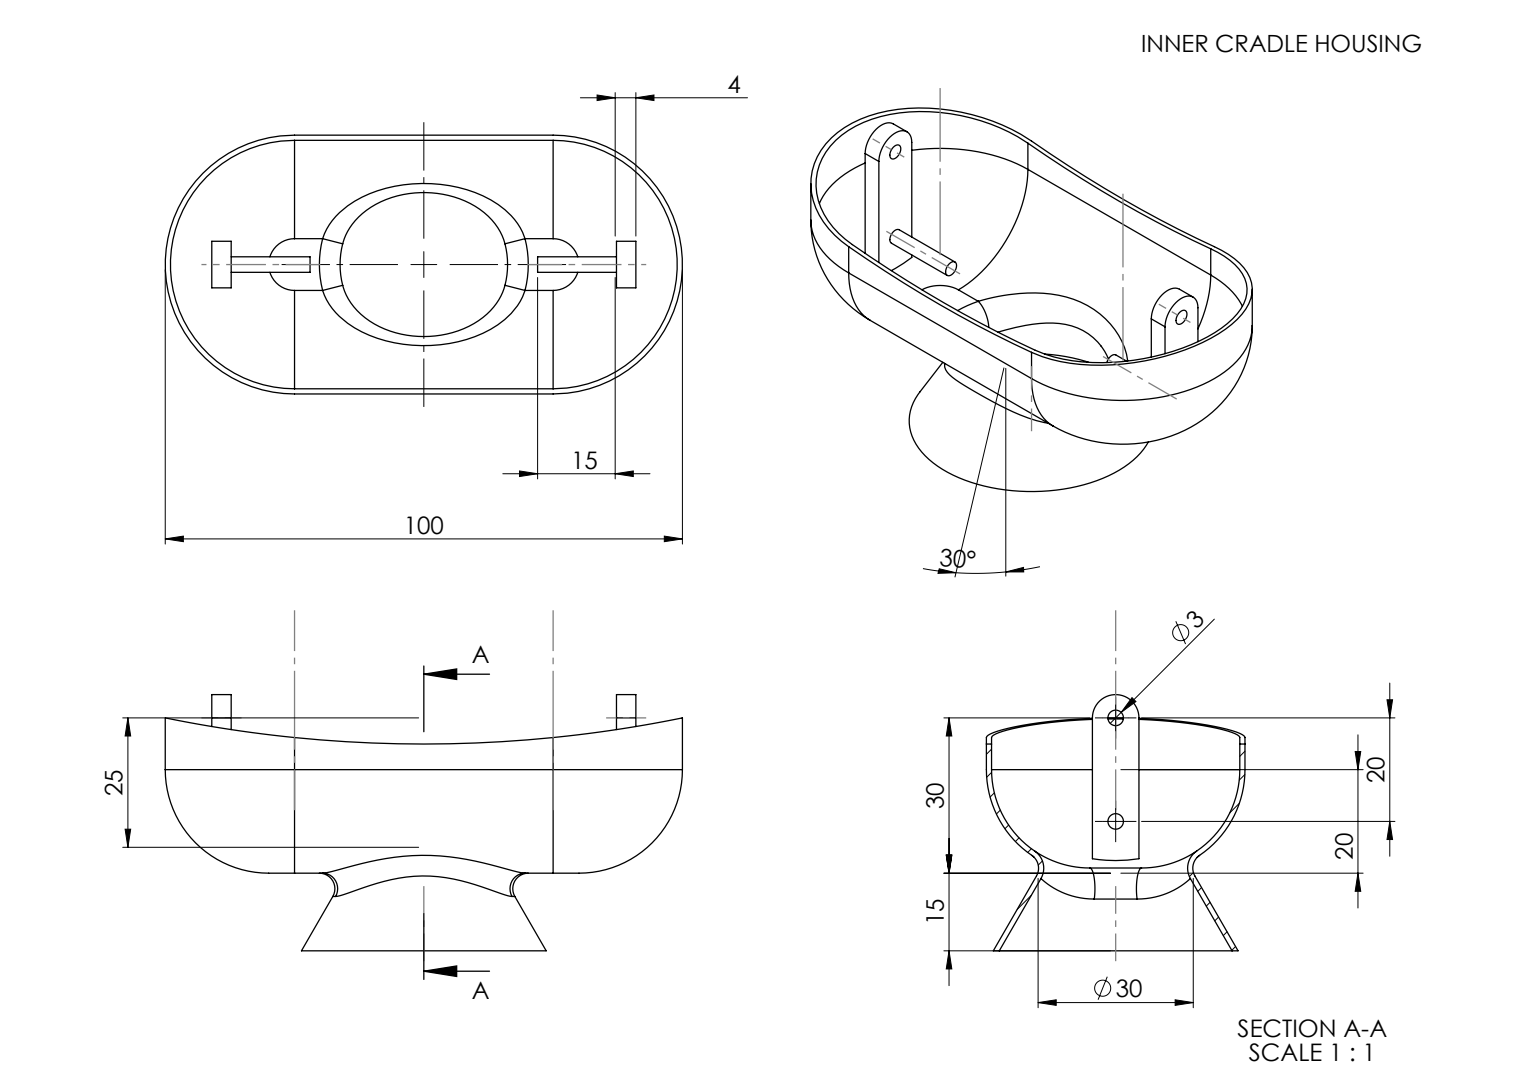
ISO-10303-21;
HEADER;
FILE_DESCRIPTION (('STEP AP214'),
    '1' );
FILE_NAME ('Inner cradle housing.step',
    '2026-10-09T15:17:24',
    ( '' ),
    ( '' ),
    'SwSTEP 2.0',
    'SolidWorks 2026',
    '' );
FILE_SCHEMA (( 'AUTOMOTIVE_DESIGN' ));
ENDSEC;

DATA;
#11=EDGE_LOOP ( 'NONE', ( #13476, #2905, #46275, #26509, #7082, #64281 ) ) ;
#18=CARTESIAN_POINT ( 'NONE',  ( -9.857630741398541119, -27.64257788600498245, 14.42778837489968424 ) ) ;
#57=CARTESIAN_POINT ( 'NONE',  ( 1.074417311476297821, -26.55384113566742599, -16.22365110280896161 ) ) ;
#110=CARTESIAN_POINT ( 'NONE',  ( 49.33927601438018229, -0.1339636383559821564, -5.724480317196142032 ) ) ;
#114=CARTESIAN_POINT ( 'NONE',  ( -38.20713125073509531, -2.115151932665340961, -21.24219930640693832 ) ) ;
#116=CARTESIAN_POINT ( 'NONE',  ( 19.56743653832046803, -28.99999999999999645, -5.000000000000000888 ) ) ;
#121=ADVANCED_FACE ( 'NONE', ( #65020 ), #19493, .F. ) ;
#146=DIRECTION ( 'NONE',  ( 1.000000000000000000, 0.000000000000000000, 0.000000000000000000 ) ) ;
#147=CARTESIAN_POINT ( 'NONE',  ( -8.315422948566315142, -32.37591480791618892, 12.77210737139424523 ) ) ;
#159=CARTESIAN_POINT ( 'NONE',  ( 14.19127861764911813, -30.11167671974727611, 5.095448428665359408 ) ) ;
#215=CARTESIAN_POINT ( 'NONE',  ( 16.21117406328132304, -34.99999999999999289, -4.142385751841744401 ) ) ;
#249=CARTESIAN_POINT ( 'NONE',  ( -41.00000000000000711, -1.694065894508600678E-18, 0.000000000000000000 ) ) ;
#284=FACE_OUTER_BOUND ( 'NONE', #48979, .T. ) ;
#285=CYLINDRICAL_SURFACE ( 'NONE', #47961, 1.500000000000000222 ) ;
#326=FACE_OUTER_BOUND ( 'NONE', #43910, .T. ) ;
#391=CARTESIAN_POINT ( 'NONE',  ( 36.99853283657033387, -2.301590494557431477, -20.84413141647362266 ) ) ;
#412=CARTESIAN_POINT ( 'NONE',  ( -5.808548865028119401, -28.57390223679843544, -12.95295593664668310 ) ) ;
#426=CARTESIAN_POINT ( 'NONE',  ( 25.00000000000000711, -30.00000000000000000, -24.00000000000000000 ) ) ;
#465=CARTESIAN_POINT ( 'NONE',  ( 15.59244419633153456, -34.16973227397373591, 7.752328951095602605 ) ) ;
#491=CARTESIAN_POINT ( 'NONE',  ( -12.26308380404417164, -33.73908083898199806, 10.29207979367737380 ) ) ;
#501=CARTESIAN_POINT ( 'NONE',  ( 10.20102756488484275, -27.72270395345634952, 14.27139701651698722 ) ) ;
#542=CARTESIAN_POINT ( 'NONE',  ( -15.05999060605171458, -34.74914171045087841, -6.965575872675125346 ) ) ;
#548=CARTESIAN_POINT ( 'NONE',  ( 15.30590914263659386, -28.05839919878968303, -10.93630420992710128 ) ) ;
#556=B_SPLINE_CURVE_WITH_KNOTS ( 'NONE', 3,
 ( #63039, #7858, #51545, #7500, #658, #6873, #56507, #1875, #12169, #47438, #22145, #2879, #2553, #27143, #33103, #23135, #10952, #42744, #32440, #62695, #52750, #63355, #20917, #31239, #5658, #61474, #28134, #48097, #22822, #32755, #17162, #37439, #43078, #12481, #18153, #53412, #27793, #25927, #47754, #17821, #57750, #46216, #33445, #17503, #15916, #37773, #53064, #2203, #7174, #36200, #38426, #41191, #22481, #38086 ),
 .UNSPECIFIED., .F., .F.,
 ( 4, 2, 2, 2, 2, 2, 2, 2, 2, 2, 2, 2, 2, 2, 2, 2, 2, 2, 2, 2, 2, 2, 2, 2, 2, 2, 4 ),
 ( 0.000000000000000000, 0.004712545709777801912, 0.007068818564666702435, 0.009425091419555603825, 0.01413763712933342048, 0.01649390998422233315, 0.01885018283911124234, 0.02356272854888905727, 0.02591900140377796299, 0.02827527425866686525, 0.03063154711355577098, 0.03180968354100022211, 0.03298781996844467324, 0.03770036567822248469, 0.04005663853311138001, 0.04123477496055583114, 0.04241291138800028920, 0.04712545709777810760, 0.04948172995266700985, 0.05183800280755592599, 0.05655054851733373744, 0.06126309422711155583, 0.06361936708200047197, 0.06597563993688937423, 0.07068818564666717874, 0.07304445850155608100, 0.07540073135644498326 ),
 .UNSPECIFIED. ) ;
#623=AXIS2_PLACEMENT_3D ( 'NONE', #44497, #64774, #4635 ) ;
#631=EDGE_CURVE ( 'NONE', #31040, #33343, #47243, .T. ) ;
#637=ORIENTED_EDGE ( 'NONE', *, *, #44495, .F. ) ;
#653=CARTESIAN_POINT ( 'NONE',  ( -17.92531974009704498, -29.71422580122558088, 8.391737566679434934 ) ) ;
#658=CARTESIAN_POINT ( 'NONE',  ( -31.19808003874556235, -3.097905286366202215, 23.19915556217947739 ) ) ;
#659=VERTEX_POINT ( 'NONE', #32553 ) ;
#690=CARTESIAN_POINT ( 'NONE',  ( -4.968020780095184108, -25.99038707641916091, -15.26464785194325913 ) ) ;
#713=LINE ( 'NONE', #60899, #29959 ) ;
#727=CARTESIAN_POINT ( 'NONE',  ( 18.66975156949926529, -29.88417193384192316, -7.188590896528729068 ) ) ;
#769=CARTESIAN_POINT ( 'NONE',  ( 49.19530910174992044, -0.1631003452855546987, 6.502801691937079021 ) ) ;
#773=CARTESIAN_POINT ( 'NONE',  ( 3.657075258475105617, -30.77912794045789724, 15.01778408663561493 ) ) ;
#799=CARTESIAN_POINT ( 'NONE',  ( 3.702144525957873356, -25.87585389521097312, 15.43847573974272613 ) ) ;
#850=CARTESIAN_POINT ( 'NONE',  ( 11.32672149592540833, -33.39346531321398714, 11.05302976539647197 ) ) ;
#856=CARTESIAN_POINT ( 'NONE',  ( 9.730232070128172595, -26.74067542416307219, -13.98809302346541372 ) ) ;
#889=EDGE_CURVE ( 'NONE', #27125, #49767, #43081, .T. ) ;
#939=VERTEX_POINT ( 'NONE', #30517 ) ;
#971=CARTESIAN_POINT ( 'NONE',  ( 41.00000000000000711, -25.03188948156373783, 4.499999999999997335 ) ) ;
#990=CARTESIAN_POINT ( 'NONE',  ( -17.07517663476617997, -28.52001404462332701, 9.261390606240922807 ) ) ;
#1000=FACE_OUTER_BOUND ( 'NONE', #53126, .T. ) ;
#1013=CARTESIAN_POINT ( 'NONE',  ( 7.856790134851108220, -26.39165916151114999, -14.61432118582568407 ) ) ;
#1036=CARTESIAN_POINT ( 'NONE',  ( 46.86486279825821555, -0.6193039491651846085, 9.927184253397724589 ) ) ;
#1044=CARTESIAN_POINT ( 'NONE',  ( 2.756135405615951955E-15, -45.00000000000000000, 22.50555349946515804 ) ) ;
#1054=CARTESIAN_POINT ( 'NONE',  ( 9.591596427418878079, -32.12122108032075118, -13.09346764506430993 ) ) ;
#1064=CARTESIAN_POINT ( 'NONE',  ( -4.348075857607831551, -31.41176936172747958, 14.02665938297152870 ) ) ;
#1072=AXIS2_PLACEMENT_3D ( 'NONE', #24249, #60472, #45192 ) ;
#1108=CIRCLE ( 'NONE', #30794, 3.999999999999999112 ) ;
#1130=CARTESIAN_POINT ( 'NONE',  ( 8.754896909465220034, -28.78086681028207749, 9.883947858767236028 ) ) ;
#1134=CYLINDRICAL_SURFACE ( 'NONE', #47965, 20.00000000000000000 ) ;
#1145=ORIENTED_EDGE ( 'NONE', *, *, #50067, .F. ) ;
#1159=CARTESIAN_POINT ( 'NONE',  ( 25.00000000000000355, -28.99999999999999645, -4.999999999999999112 ) ) ;
#1164=DIRECTION ( 'NONE',  ( 0.000000000000000000, -0.000000000000000000, 1.000000000000000000 ) ) ;
#1172=CIRCLE ( 'NONE', #59553, 1.500000000000000222 ) ;
#1234=VECTOR ( 'NONE', #2454, 1000.000000000000000 ) ;
#1256=FACE_BOUND ( 'NONE', #34167, .T. ) ;
#1266=DIRECTION ( 'NONE',  ( 0.000000000000000000, 0.000000000000000000, 1.000000000000000000 ) ) ;
#1314=ORIENTED_EDGE ( 'NONE', *, *, #9225, .T. ) ;
#1316=CARTESIAN_POINT ( 'NONE',  ( -19.56743653832047158, -33.00000000000000000, 5.000000000000000888 ) ) ;
#1323=EDGE_LOOP ( 'NONE', ( #39107, #2329, #36527, #17256 ) ) ;
#1346=ORIENTED_EDGE ( 'NONE', *, *, #6034, .T. ) ;
#1350=CARTESIAN_POINT ( 'NONE',  ( 9.722110222095126986, -26.73349363795548328, -14.00621188957225272 ) ) ;
#1357=CARTESIAN_POINT ( 'NONE',  ( -19.56743653832047514, -30.00000000000000000, 5.000000000000000888 ) ) ;
#1395=CARTESIAN_POINT ( 'NONE',  ( 19.43600551875691451, -29.99999999999999645, -5.447264023289523749 ) ) ;
#1397=ORIENTED_EDGE ( 'NONE', *, *, #11958, .F. ) ;
#1476=CARTESIAN_POINT ( 'NONE',  ( 3.024435290549866817, -27.93754772256033192, 12.30283293119135202 ) ) ;
#1547=EDGE_CURVE ( 'NONE', #54224, #31440, #12444, .T. ) ;
#1551=LINE ( 'NONE', #37087, #27003 ) ;
#1610=CARTESIAN_POINT ( 'NONE',  ( -49.33927601438018939, -0.1339636383559742183, 5.724480317196145585 ) ) ;
#1683=CARTESIAN_POINT ( 'NONE',  ( -0.4967434119545894866, -25.72578597719286364, -15.66300405139958407 ) ) ;
#1702=CARTESIAN_POINT ( 'NONE',  ( 48.61333473403966821, -0.2789806315675412152, 4.308813575818149388 ) ) ;
#1709=ADVANCED_FACE ( 'NONE', ( #31357 ), #52315, .T. ) ;
#1718=CARTESIAN_POINT ( 'NONE',  ( 9.992127424267872371, -32.24574823824523406, -12.88148438038769150 ) ) ;
#1725=CARTESIAN_POINT ( 'NONE',  ( 16.21117406328131594, -35.00000000000000000, -4.142385751841773711 ) ) ;
#1730=FACE_OUTER_BOUND ( 'NONE', #16630, .T. ) ;
#1736=EDGE_CURVE ( 'NONE', #3747, #26969, #6009, .T. ) ;
#1788=DIRECTION ( 'NONE',  ( -0.9688695217174486674, 0.000000000000000000, -0.2475719085175094036 ) ) ;
#1792=CARTESIAN_POINT ( 'NONE',  ( 5.926183177043330197, -31.73296902231061978, 13.63811545878544607 ) ) ;
#1799=EDGE_CURVE ( 'NONE', #65150, #23145, #39949, .T. ) ;
#1810=DIRECTION ( 'NONE',  ( 0.000000000000000000, 1.000000000000000000, 0.000000000000000000 ) ) ;
#1813=DIRECTION ( 'NONE',  ( 0.000000000000000000, 0.000000000000000000, -1.000000000000000000 ) ) ;
#1827=EDGE_CURVE ( 'NONE', #7333, #31040, #33603, .T. ) ;
#1875=CARTESIAN_POINT ( 'NONE',  ( -35.62380706382417372, -2.504225566391070856, 21.57767586339570443 ) ) ;
#1923=CARTESIAN_POINT ( 'NONE',  ( -12.81094353615575088, -29.07674955874293943, -3.635823793966369788 ) ) ;
#2014=CARTESIAN_POINT ( 'NONE',  ( 31.24126863879125438, -3.096129103239020797, 23.22707964006411530 ) ) ;
#2031=CARTESIAN_POINT ( 'NONE',  ( 8.782331025771476618, -31.88110954670732866, -13.48440172003491178 ) ) ;
#2037=DIRECTION ( 'NONE',  ( 0.000000000000000000, 0.000000000000000000, 1.000000000000000000 ) ) ;
#2072=CARTESIAN_POINT ( 'NONE',  ( 19.24109636373441390, -29.98159021036885363, -5.977446804020350335 ) ) ;
#2100=DIRECTION ( 'NONE',  ( 0.000000000000000000, 0.000000000000000000, 1.000000000000000000 ) ) ;
#2108=CARTESIAN_POINT ( 'NONE',  ( 13.74768401152558894, -27.65692779101644305, 12.04119239038937117 ) ) ;
#2140=DIRECTION ( 'NONE',  ( 0.000000000000000000, -1.000000000000000000, 0.000000000000000000 ) ) ;
#2158=LINE ( 'NONE', #52714, #51393 ) ;
#2178=VECTOR ( 'NONE', #11059, 1000.000000000000000 ) ;
#2201=CARTESIAN_POINT ( 'NONE',  ( -15.83540182711247191, -34.24586518154816872, 7.348477566591424370 ) ) ;
#2203=CARTESIAN_POINT ( 'NONE',  ( -32.73308617475133531, -2.903166307960748593, -22.77405829473930865 ) ) ;
#2252=CIRCLE ( 'NONE', #10729, 1.500000000000000222 ) ;
#2259=CARTESIAN_POINT ( 'NONE',  ( -12.58725039716645000, -33.86007533429943095, -10.00564543523592320 ) ) ;
#2269=VERTEX_POINT ( 'NONE', #41398 ) ;
#2273=AXIS2_PLACEMENT_3D ( 'NONE', #3939, #24202, #8262 ) ;
#2295=CARTESIAN_POINT ( 'NONE',  ( -14.80332308495361815, -33.90539544391017301, -8.876538241604327695 ) ) ;
#2310=FACE_BOUND ( 'NONE', #52616, .T. ) ;
#2329=ORIENTED_EDGE ( 'NONE', *, *, #24038, .F. ) ;
#2344=AXIS2_PLACEMENT_3D ( 'NONE', #27897, #6645, #37868 ) ;
#2349=CARTESIAN_POINT ( 'NONE',  ( -8.868684597663976987, -31.89901926473304883, 13.46243262195112678 ) ) ;
#2361=CARTESIAN_POINT ( 'NONE',  ( 25.79281180259795292, -3.718204414137759262, 24.00000000000000355 ) ) ;
#2384=ORIENTED_EDGE ( 'NONE', *, *, #27450, .F. ) ;
#2421=CARTESIAN_POINT ( 'NONE',  ( 9.836964722002395689, -27.64452029744604644, -14.41904541651817873 ) ) ;
#2441=ORIENTED_EDGE ( 'NONE', *, *, #38364, .T. ) ;
#2454=DIRECTION ( 'NONE',  ( 6.123233995736778362E-17, -0.8660254037844380415, 0.5000000000000009992 ) ) ;
#2553=CARTESIAN_POINT ( 'NONE',  ( -41.38732981120779186, -1.602042930228848583, 17.55180477253565030 ) ) ;
#2561=AXIS2_PLACEMENT_3D ( 'NONE', #19143, #40066, #50410 ) ;
#2583=DIRECTION ( 'NONE',  ( -1.000000000000000000, 0.000000000000000000, 0.000000000000000000 ) ) ;
#2611=CARTESIAN_POINT ( 'NONE',  ( -13.20530710592869283, -34.09051099065911217, -9.405657446765959051 ) ) ;
#2646=ORIENTED_EDGE ( 'NONE', *, *, #13071, .F. ) ;
#2649=ORIENTED_EDGE ( 'NONE', *, *, #13071, .T. ) ;
#2723=ORIENTED_EDGE ( 'NONE', *, *, #63965, .F. ) ;
#2766=CARTESIAN_POINT ( 'NONE',  ( 2.022082860508893187, -26.59007814299271999, -16.17076096363556914 ) ) ;
#2786=VECTOR ( 'NONE', #40970, 1000.000000000000000 ) ;
#2839=CARTESIAN_POINT ( 'NONE',  ( 16.93394556191337230, -34.50000000000000000, 4.811904876957209254 ) ) ;
#2865=DIRECTION ( 'NONE',  ( 0.000000000000000000, 0.000000000000000000, 1.000000000000000000 ) ) ;
#2875=CARTESIAN_POINT ( 'NONE',  ( -7.049735699850023352, -28.78059498260736504, 12.46475915493964415 ) ) ;
#2879=CARTESIAN_POINT ( 'NONE',  ( -40.80553070818748296, -1.699139512677864561, 18.07784515657014168 ) ) ;
#2905=ORIENTED_EDGE ( 'NONE', *, *, #10978, .T. ) ;
#2914=CARTESIAN_POINT ( 'NONE',  ( -49.59714883329487378, -0.08190040965286676800, -4.488761805454715592 ) ) ;
#2956=DIRECTION ( 'NONE',  ( 0.000000000000000000, 0.000000000000000000, 1.000000000000000000 ) ) ;
#2963=ORIENTED_EDGE ( 'NONE', *, *, #9225, .F. ) ;
#2970=FACE_OUTER_BOUND ( 'NONE', #29494, .T. ) ;
#2994=DIRECTION ( 'NONE',  ( -0.000000000000000000, -1.000000000000000000, -0.000000000000000000 ) ) ;
#3000=CARTESIAN_POINT ( 'NONE',  ( 16.78995969943013478, -34.48221411999237773, -5.258039666742740259 ) ) ;
#3020=ORIENTED_EDGE ( 'NONE', *, *, #57969, .F. ) ;
#3040=ORIENTED_EDGE ( 'NONE', *, *, #50249, .F. ) ;
#3123=EDGE_CURVE ( 'NONE', #46997, #34941, #52958, .T. ) ;
#3139=AXIS2_PLACEMENT_3D ( 'NONE', #59983, #46975, #61929 ) ;
#3193=CARTESIAN_POINT ( 'NONE',  ( -6.227954140665750593, -28.64022186353238553, 12.80077302199559419 ) ) ;
#3209=CARTESIAN_POINT ( 'NONE',  ( 25.00000000000000355, -9.999999999999998224, 1.530808498934191521E-15 ) ) ;
#3214=DIRECTION ( 'NONE',  ( 0.000000000000000000, 0.000000000000000000, -1.000000000000000000 ) ) ;
#3223=DIRECTION ( 'NONE',  ( -1.000000000000000000, -0.000000000000000000, 0.000000000000000000 ) ) ;
#3248=CARTESIAN_POINT ( 'NONE',  ( 4.261270162784661863, -31.40576903066106240, -14.03034928007075344 ) ) ;
#3255=LINE ( 'NONE', #17561, #52176 ) ;
#3280=DIRECTION ( 'NONE',  ( 1.000000000000000000, -0.000000000000000000, -0.000000000000000000 ) ) ;
#3285=CYLINDRICAL_SURFACE ( 'NONE', #63068, 1.500000000000000444 ) ;
#3299=AXIS2_PLACEMENT_3D ( 'NONE', #41370, #36726, #26420 ) ;
#3329=CARTESIAN_POINT ( 'NONE',  ( 14.80527133490444314, -33.90607016887765468, -8.874040421132026069 ) ) ;
#3387=ORIENTED_EDGE ( 'NONE', *, *, #9032, .F. ) ;
#3397=AXIS2_PLACEMENT_3D ( 'NONE', #54729, #14943, #35571 ) ;
#3414=CARTESIAN_POINT ( 'NONE',  ( 19.56743653832047158, -30.00000000000000000, -5.000000000000000888 ) ) ;
#3444=AXIS2_PLACEMENT_3D ( 'NONE', #65419, #19888, #55799 ) ;
#3457=B_SPLINE_CURVE_WITH_KNOTS ( 'NONE', 3,
 ( #15365, #6066, #45617, #51294, #35307, #41938, #1064, #56250, #6381, #10692, #46295, #55620, #41613, #61900, #46943, #16359, #36633, #56937, #11355, #5077, #20689, #50952, #5400, #21683, #35639, #62225 ),
 .UNSPECIFIED., .F., .F.,
 ( 4, 2, 2, 2, 2, 2, 2, 2, 2, 2, 2, 2, 4 ),
 ( 0.02137397820462155415, 0.02270922547143531048, 0.02404447273824906334, 0.02671496727187657599, 0.02805021453869033232, 0.02938546180550408865, 0.03205595633913160825, 0.03472645087275912090, 0.03606169813957287723, 0.03739694540638663356, 0.03873219267320038989, 0.04006743994001414622, 0.04273793447364165887 ),
 .UNSPECIFIED. ) ;
#3533=VECTOR ( 'NONE', #14513, 1000.000000000000000 ) ;
#3536=CARTESIAN_POINT ( 'NONE',  ( -11.13200843151504849, -27.92871652161695550, 13.87829993151233943 ) ) ;
#3594=CARTESIAN_POINT ( 'NONE',  ( -0.4223990570890304164, -27.81390085543024426, -12.58355210400658564 ) ) ;
#3606=CYLINDRICAL_SURFACE ( 'NONE', #18532, 4.500000000000000888 ) ;
#3650=CARTESIAN_POINT ( 'NONE',  ( -16.66082797316812503, -33.00000000000000000, 4.257284274447473926 ) ) ;
#3718=CARTESIAN_POINT ( 'NONE',  ( -15.84367078532069861, -34.24835312396456999, -7.333865081863226720 ) ) ;
#3747=VERTEX_POINT ( 'NONE', #11496 ) ;
#3768=EDGE_LOOP ( 'NONE', ( #43729, #12929, #2649, #45049, #41030, #14374, #10511 ) ) ;
#3781=CARTESIAN_POINT ( 'NONE',  ( 19.56743653832047869, -28.99999999999999289, 4.999999999999984901 ) ) ;
#3823=CARTESIAN_POINT ( 'NONE',  ( 25.00000000000000711, -3.797884998337192286, -25.00000000000000000 ) ) ;
#3853=ADVANCED_FACE ( 'NONE', ( #7484 ), #33087, .F. ) ;
#3859=CARTESIAN_POINT ( 'NONE',  ( 2.128776824815523216, -26.59425375115992907, 16.16470972310802523 ) ) ;
#3889=VERTEX_POINT ( 'NONE', #38408 ) ;
#3902=CARTESIAN_POINT ( 'NONE',  ( -11.13200843151504849, -27.03228069553586010, -13.43438493493725616 ) ) ;
#3939=CARTESIAN_POINT ( 'NONE',  ( -19.56743653832047158, -33.00000000000000000, 5.000000000000000888 ) ) ;
#3970=CARTESIAN_POINT ( 'NONE',  ( 16.25676674326364335, -34.36623312464833191, -6.550321452248093479 ) ) ;
#3978=CARTESIAN_POINT ( 'NONE',  ( -17.05023968204110929, -34.50000000000000000, 4.356789313881321846 ) ) ;
#3996=CARTESIAN_POINT ( 'NONE',  ( -16.66082797316812503, -33.00000000000000000, -4.257284274447473926 ) ) ;
#4012=ADVANCED_BREP_SHAPE_REPRESENTATION ( '', ( #7246, #24966 ), #5855 ) ;
#4047=CARTESIAN_POINT ( 'NONE',  ( 37.25000000000000711, 5.493969937218003549E-16, -4.500000000000000888 ) ) ;
#4069=ORIENTED_EDGE ( 'NONE', *, *, #6633, .F. ) ;
#4077=CARTESIAN_POINT ( 'NONE',  ( -6.227954140666513538, -28.64022186353147248, -12.80077302199831557 ) ) ;
#4101=FACE_OUTER_BOUND ( 'NONE', #23994, .T. ) ;
#4128=B_SPLINE_CURVE_WITH_KNOTS ( 'NONE', 3,
 ( #3823, #53694, #19086, #44658, #13113, #23417, #39353, #54680, #29382, #24389, #64945, #39692, #59987, #14405, #34681, #54978, #60295, #56641, #46329, #25712, #65286, #26047, #5780, #110, #40670, #20066, #30677, #50986, #35671, #20392, #45011, #25062, #31022, #769, #56285, #14719, #45657, #55306, #5109, #10089, #65591, #60967, #34998, #31352, #45331, #50349, #9749, #15400, #40328, #30036, #50665, #21031, #51655, #4797 ),
 .UNSPECIFIED., .F., .F.,
 ( 4, 2, 2, 2, 2, 2, 2, 2, 2, 2, 2, 2, 2, 2, 2, 2, 2, 2, 2, 2, 2, 2, 2, 2, 2, 2, 4 ),
 ( 0.000000000000000000, 0.004909564951003675057, 0.007364347426505513453, 0.009819129902007351848, 0.01472869485301103037, 0.01718347732851286530, 0.01963825980401470023, 0.02454782475501837702, 0.02700260723052020501, 0.02945738970602204340, 0.03191217218152387486, 0.03313956341927479232, 0.03436695465702570979, 0.03927651960802938658, 0.04173130208353122844, 0.04295869332128214590, 0.04418608455903306337, 0.04909564951003673322, 0.05155043198553856121, 0.05400521446104038920, 0.05891477941204405905, 0.06382434436304772196, 0.06627912683854955689, 0.06873390931405140569, 0.07364347426505506167, 0.07609825674055691047, 0.07855303921605873152 ),
 .UNSPECIFIED. ) ;
#4154=CARTESIAN_POINT ( 'NONE',  ( -15.30016555129190792, -28.05832310202213620, 10.91616026484521385 ) ) ;
#4166=CARTESIAN_POINT ( 'NONE',  ( -5.813762929211682362, -31.14503107145061378, 14.54886001617130553 ) ) ;
#4212=CARTESIAN_POINT ( 'NONE',  ( 2.128776824815522772, -25.76454106360162299, -15.60647423695309222 ) ) ;
#4231=CARTESIAN_POINT ( 'NONE',  ( 41.00000000000000711, -1.694065894508793271E-18, 4.500000000000001776 ) ) ;
#4261=FACE_OUTER_BOUND ( 'NONE', #54065, .T. ) ;
#4339=DIRECTION ( 'NONE',  ( 0.000000000000000000, 0.000000000000000000, 1.000000000000000000 ) ) ;
#4345=CARTESIAN_POINT ( 'NONE',  ( -8.868684597672961800, -31.89901926473567784, -13.46243262194695944 ) ) ;
#4347=FACE_BOUND ( 'NONE', #55657, .T. ) ;
#4363=ORIENTED_EDGE ( 'NONE', *, *, #44501, .T. ) ;
#4370=CARTESIAN_POINT ( 'NONE',  ( -0.5028117989624503181, -26.55343892596427224, 16.22424428316958256 ) ) ;
#4384=CARTESIAN_POINT ( 'NONE',  ( -4.047649113456406766, -26.73415408998408083, -15.95376587162192905 ) ) ;
#4390=AXIS2_PLACEMENT_3D ( 'NONE', #4757, #35299, #32194 ) ;
#4414=ORIENTED_EDGE ( 'NONE', *, *, #59041, .T. ) ;
#4416=CARTESIAN_POINT ( 'NONE',  ( 4.958255736528643709, -30.98164499407788242, -14.76282592124297288 ) ) ;
#4423=CARTESIAN_POINT ( 'NONE',  ( -41.00000000000000711, -1.694065894508600678E-18, 0.000000000000000000 ) ) ;
#4427=AXIS2_PLACEMENT_3D ( 'NONE', #65603, #61603, #11088 ) ;
#4465=CARTESIAN_POINT ( 'NONE',  ( 0.000000000000000000, -33.00000000000000000, 0.000000000000000000 ) ) ;
#4468=CARTESIAN_POINT ( 'NONE',  ( 10.04668509498937645, -32.26295471732144193, 12.85148783289558239 ) ) ;
#4496=CARTESIAN_POINT ( 'NONE',  ( -15.98984497772178770, -34.99999999818471963, 5.008554314762531767 ) ) ;
#4506=CARTESIAN_POINT ( 'NONE',  ( 16.03117610287102579, -29.21144266226587760, 10.60889071582655241 ) ) ;
#4551=CARTESIAN_POINT ( 'NONE',  ( -4.348075857621052087, -31.41176936172981726, -14.02665938296879844 ) ) ;
#4552=AXIS2_PLACEMENT_3D ( 'NONE', #25407, #56318, #146 ) ;
#4557=CARTESIAN_POINT ( 'NONE',  ( -0.4156926711315701573, -31.03628804997841684, -14.44394305974772408 ) ) ;
#4569=VERTEX_POINT ( 'NONE', #57238 ) ;
#4586=ORIENTED_EDGE ( 'NONE', *, *, #63632, .F. ) ;
#4587=DIRECTION ( 'NONE',  ( 1.000000000000000000, -0.000000000000000000, -0.000000000000000000 ) ) ;
#4635=DIRECTION ( 'NONE',  ( 0.000000000000000000, 0.000000000000000000, 1.000000000000000000 ) ) ;
#4641=ORIENTED_EDGE ( 'NONE', *, *, #40737, .F. ) ;
#4659=DIRECTION ( 'NONE',  ( 0.000000000000000000, 0.000000000000000000, 1.000000000000000000 ) ) ;
#4671=CARTESIAN_POINT ( 'NONE',  ( -15.69195845145067736, -33.00000000000000000, 4.009712365929964051 ) ) ;
#4694=CARTESIAN_POINT ( 'NONE',  ( -0.4967434119545920956, -25.72578597719286719, 15.66300405139958407 ) ) ;
#4755=CARTESIAN_POINT ( 'NONE',  ( -2.112161198360044789, -26.60281475960666953, -16.15113466974405654 ) ) ;
#4757=CARTESIAN_POINT ( 'NONE',  ( 19.56743653832047514, -33.00000000000000000, 5.000000000000001776 ) ) ;
#4790=ADVANCED_FACE ( 'NONE', ( #326 ), #43690, .F. ) ;
#4797=CARTESIAN_POINT ( 'NONE',  ( 25.00000000000000355, -3.797884998337192286, 24.99999999999999289 ) ) ;
#4822=FACE_OUTER_BOUND ( 'NONE', #40884, .T. ) ;
#4825=CARTESIAN_POINT ( 'NONE',  ( -12.31125281582930064, -29.30934768819192371, 5.548768499314465252 ) ) ;
#4836=CARTESIAN_POINT ( 'NONE',  ( 4.532733354134460768, -28.39821948934986651, 13.34103783736875215 ) ) ;
#4872=CARTESIAN_POINT ( 'NONE',  ( 13.23110845410259451, -34.10188054478469155, 9.409930202772073926 ) ) ;
#4880=CARTESIAN_POINT ( 'NONE',  ( 14.81496943876074290, -34.66917994667981162, -7.369609160621835464 ) ) ;
#4905=ORIENTED_EDGE ( 'NONE', *, *, #52253, .F. ) ;
#4934=B_SPLINE_CURVE_WITH_KNOTS ( 'NONE', 3,
 ( #13330, #48593, #43572, #63855, #33616, #990, #61824, #30263, #16279, #60852, #19950, #26257, #15292, #35570, #50235, #50560, #15927, #36211, #41203, #14941, #35233, #50877, #4694, #40559, #9629, #55197, #29927, #55536, #9984, #5322, #5004, #55864, #56177, #24955, #10295, #15609, #30572, #10613, #65805, #25597, #45228, #45891, #61488, #20279, #25262, #30899 ),
 .UNSPECIFIED., .F., .F.,
 ( 4, 2, 2, 2, 2, 2, 2, 2, 2, 2, 2, 2, 2, 2, 2, 2, 2, 2, 2, 2, 2, 2, 4 ),
 ( 0.000000000000000000, 0.002978983955370559291, 0.004468475933055836118, 0.005957967910741112511, 0.007447459888426388036, 0.008936951866111665296, 0.01191593582148221461, 0.01489491977685276219, 0.01787390373222331325, 0.02085288768759386083, 0.02234237966527913288, 0.02383187164296440841, 0.02681085559833495946, 0.02830034757602023499, 0.02978983955370551051, 0.03276882350907605462, 0.03574780746444660567, 0.03872679141981715673, 0.04170577537518770778, 0.04319526735287298330, 0.04468475933055825883, 0.04617425130824354129, 0.04766374328592882376 ),
 .UNSPECIFIED. ) ;
#4999=CARTESIAN_POINT ( 'NONE',  ( 2.897545437445938920E-15, -45.00000000000000000, 23.66025403784440684 ) ) ;
#5004=CARTESIAN_POINT ( 'NONE',  ( 7.856790134851106444, -26.39165916151114288, 14.61432118582567874 ) ) ;
#5024=CARTESIAN_POINT ( 'NONE',  ( -10.77421046970567353, -27.84620353580639573, 14.04190754122876506 ) ) ;
#5066=CARTESIAN_POINT ( 'NONE',  ( 5.786001662379491428, -26.94056086434354924, -15.63186719136363756 ) ) ;
#5077=CARTESIAN_POINT ( 'NONE',  ( -14.08345347783795987, -34.41374607521820650, 8.401505689979551050 ) ) ;
#5101=DIRECTION ( 'NONE',  ( 0.000000000000000000, 0.000000000000000000, -1.000000000000000000 ) ) ;
#5109=CARTESIAN_POINT ( 'NONE',  ( 46.22120612461745282, -0.7415077656649037285, 13.24100464050679449 ) ) ;
#5111=CARTESIAN_POINT ( 'NONE',  ( -26.64924965067720208, -3.627973872667547450, -24.95916750106484372 ) ) ;
#5141=CARTESIAN_POINT ( 'NONE',  ( -13.72965000697191584, -27.65230582893893896, 12.05355732046426809 ) ) ;
#5152=CARTESIAN_POINT ( 'NONE',  ( 18.88852658721791045, -29.92669765328983544, 6.766054962673704765 ) ) ;
#5199=CARTESIAN_POINT ( 'NONE',  ( 18.88852658721791045, -28.93036277062534012, -6.677752214540050524 ) ) ;
#5223=EDGE_CURVE ( 'NONE', #51364, #52741, #20993, .T. ) ;
#5322=CARTESIAN_POINT ( 'NONE',  ( 6.904443316226201333, -26.24011843744384009, 14.86481251185163366 ) ) ;
#5349=CARTESIAN_POINT ( 'NONE',  ( 10.63650944684269639, -26.92414420718871071, -13.64813004266018481 ) ) ;
#5356=AXIS2_PLACEMENT_3D ( 'NONE', #8494, #45304, #40969 ) ;
#5368=ORIENTED_EDGE ( 'NONE', *, *, #13546, .F. ) ;
#5371=CARTESIAN_POINT ( 'NONE',  ( 37.67868074218839070, -2.196220884325986500, 20.39261666198438405 ) ) ;
#5391=CARTESIAN_POINT ( 'NONE',  ( -0.8948477690460417966, -30.54755392045676032, -15.29677453898885808 ) ) ;
#5398=ORIENTED_EDGE ( 'NONE', *, *, #7792, .T. ) ;
#5400=CARTESIAN_POINT ( 'NONE',  ( -15.05999060605047646, -34.74914171045048050, 6.965575872677295166 ) ) ;
#5458=ORIENTED_EDGE ( 'NONE', *, *, #50357, .T. ) ;
#5473=CIRCLE ( 'NONE', #37298, 4.500000000000000888 ) ;
#5480=CARTESIAN_POINT ( 'NONE',  ( -9.974301738911194093, -29.01869747443698344, 8.904338584474110974 ) ) ;
#5489=B_SPLINE_CURVE_WITH_KNOTS ( 'NONE', 3,
 ( #3414, #32321, #2072, #33317, #7059, #22341, #17709, #8062, #43956, #64230, #52942, #43604, #58265, #42609, #63897, #2421, #22698, #32628, #42962, #12686, #7725, #28012, #63555, #2766, #43278, #44929, #39278, #20311, #50593, #4384, #65211, #29310, #19985, #40255, #19346, #19681, #14008, #55576, #64539, #55232, #60222, #33959, #54607, #44268, #19012, #29961, #50267, #60543 ),
 .UNSPECIFIED., .F., .F.,
 ( 4, 2, 2, 2, 2, 2, 2, 2, 2, 2, 2, 2, 2, 2, 2, 2, 2, 2, 2, 2, 2, 2, 2, 4 ),
 ( 1.262897753262583006E-17, 0.001542731309856127829, 0.003085462619712243081, 0.004628193929568360718, 0.006170925239424478355, 0.009256387859136719701, 0.01234185047884896538, 0.01388458178870508909, 0.01542731309856121280, 0.01851277571827345328, 0.02005550702812957525, 0.02159823833798569723, 0.02468370095769793424, 0.02622643226755405621, 0.02776916357741017818, 0.03085462619712241866, 0.03394008881683466261, 0.03702555143654689962, 0.04011101405625914357, 0.04165374536611526207, 0.04319647667597138752, 0.04473920798582751296, 0.04628193929568363840, 0.04936740191539588929 ),
 .UNSPECIFIED. ) ;
#5493=CARTESIAN_POINT ( 'NONE',  ( 9.730232070128172595, -27.62176360438249390, 14.46115055101565972 ) ) ;
#5542=CARTESIAN_POINT ( 'NONE',  ( 19.56743653832047869, -28.99999999999999289, -4.999999999999984901 ) ) ;
#5575=ORIENTED_EDGE ( 'NONE', *, *, #32647, .F. ) ;
#5607=ORIENTED_EDGE ( 'NONE', *, *, #57749, .F. ) ;
#5626=FACE_OUTER_BOUND ( 'NONE', #43588, .T. ) ;
#5658=CARTESIAN_POINT ( 'NONE',  ( -48.45393016956177235, -0.3105270330721054961, 5.105971556042225856 ) ) ;
#5665=AXIS2_PLACEMENT_3D ( 'NONE', #36266, #25644, #56569 ) ;
#5692=CARTESIAN_POINT ( 'NONE',  ( -37.25000000000000711, -27.21021009056489248, -4.500000000000000888 ) ) ;
#5694=DIRECTION ( 'NONE',  ( 0.9688695217174486674, 5.204170427930422072E-15, -0.2475719085175099865 ) ) ;
#5715=CARTESIAN_POINT ( 'NONE',  ( 46.51586683006346590, -0.6857498399870713968, -10.66240463596387400 ) ) ;
#5727=EDGE_CURVE ( 'NONE', #62996, #52558, #51712, .T. ) ;
#5735=CARTESIAN_POINT ( 'NONE',  ( 7.125164966884262263, -31.43290117443645926, -14.16047883281914110 ) ) ;
#5780=CARTESIAN_POINT ( 'NONE',  ( 49.13724917365554745, -0.1745483773780858450, -6.524050439336988028 ) ) ;
#5819=CARTESIAN_POINT ( 'NONE',  ( 9.461050110694847248, -32.74574823825055603, 12.19700847635464669 ) ) ;
#5830=CARTESIAN_POINT ( 'NONE',  ( 7.085269882676145770, -28.78331678330111387, 12.46778293907355994 ) ) ;
#5855=( GEOMETRIC_REPRESENTATION_CONTEXT ( 3 ) GLOBAL_UNCERTAINTY_ASSIGNED_CONTEXT ( ( #58286 ) ) GLOBAL_UNIT_ASSIGNED_CONTEXT ( ( #42479, #52816, #43471 ) ) REPRESENTATION_CONTEXT ( 'NONE', 'WORKASPACE' ) );
#5878=CARTESIAN_POINT ( 'NONE',  ( 11.77510182854060439, -29.30972061338851375, -6.669332763618045057 ) ) ;
#5906=LINE ( 'NONE', #30159, #3533 ) ;
#5907=ADVANCED_FACE ( 'NONE', ( #4101 ), #13731, .T. ) ;
#5917=DIRECTION ( 'NONE',  ( 0.000000000000000000, 0.000000000000000000, 1.000000000000000000 ) ) ;
#5924=CYLINDRICAL_SURFACE ( 'NONE', #7566, 20.00000000000000000 ) ;
#5935=FACE_OUTER_BOUND ( 'NONE', #35780, .T. ) ;
#5957=ORIENTED_EDGE ( 'NONE', *, *, #38142, .T. ) ;
#5990=CARTESIAN_POINT ( 'NONE',  ( -15.30016555129098599, -29.00876116002302396, -11.22753712089058808 ) ) ;
#6009=CIRCLE ( 'NONE', #29320, 17.59807621135332312 ) ;
#6023=( NAMED_UNIT ( * ) SI_UNIT ( $, .STERADIAN. ) SOLID_ANGLE_UNIT ( ) );
#6034=EDGE_CURVE ( 'NONE', #3889, #38752, #30659, .T. ) ;
#6035=APPLICATION_CONTEXT ( 'automotive_design' ) ;
#6044=CARTESIAN_POINT ( 'NONE',  ( 48.17199526896421702, -0.3660652840184965284, -6.262213226250246123 ) ) ;
#6058=CARTESIAN_POINT ( 'NONE',  ( 16.03117610287102579, -29.21144266226587760, -10.60889071582655241 ) ) ;
#6066=CARTESIAN_POINT ( 'NONE',  ( -0.4370662499787615340, -31.03649492335484439, 14.44372008463347079 ) ) ;
#6130=CARTESIAN_POINT ( 'NONE',  ( 1.074417311476293158, -25.72614907888524982, 15.66246854766675156 ) ) ;
#6138=ORIENTED_EDGE ( 'NONE', *, *, #35252, .T. ) ;
#6180=CARTESIAN_POINT ( 'NONE',  ( 15.63877597542616016, -34.91516792956262805, 5.826750174075395527 ) ) ;
#6224=ORIENTED_EDGE ( 'NONE', *, *, #37212, .F. ) ;
#6261=CARTESIAN_POINT ( 'NONE',  ( -41.46388549984529703, -1.589384660823694562, 18.83126657550987559 ) ) ;
#6299=CARTESIAN_POINT ( 'NONE',  ( -16.47895549814540317, -34.42947327577542893, -6.127516784536645389 ) ) ;
#6321=DIRECTION ( 'NONE',  ( 1.000000000000000000, -0.000000000000000000, 0.000000000000000000 ) ) ;
#6332=CARTESIAN_POINT ( 'NONE',  ( -12.41459945261391162, -27.32694502519497348, -12.80960016232523202 ) ) ;
#6337=CARTESIAN_POINT ( 'NONE',  ( 41.00000000000000711, 5.493969937218003549E-16, -4.500000000000000888 ) ) ;
#6356=CARTESIAN_POINT ( 'NONE',  ( 43.04762206662383761, -1.319502909267364243, -15.89732852394791784 ) ) ;
#6363=AXIS2_PLACEMENT_3D ( 'NONE', #59574, #39936, #34293 ) ;
#6373=CARTESIAN_POINT ( 'NONE',  ( 14.42557999471933705, -30.05477271089583269, -4.241434648442556465 ) ) ;
#6381=CARTESIAN_POINT ( 'NONE',  ( -6.008663266758395238, -31.76136623419596106, 13.60005156548239036 ) ) ;
#6441=CARTESIAN_POINT ( 'NONE',  ( -37.25000000000000711, -27.21021009056489248, -4.500000000000000888 ) ) ;
#6447=CARTESIAN_POINT ( 'NONE',  ( -2.167161191928854258, -27.87656208324061069, 12.44306432472098756 ) ) ;
#6473=DIRECTION ( 'NONE',  ( -1.000000000000000000, 0.000000000000000000, -0.000000000000000000 ) ) ;
#6495=CARTESIAN_POINT ( 'NONE',  ( -40.99999999999999289, -25.49182303066451993, -1.512869109757708941 ) ) ;
#6549=DIRECTION ( 'NONE',  ( 0.000000000000000000, 1.000000000000000000, 0.000000000000000000 ) ) ;
#6591=CARTESIAN_POINT ( 'NONE',  ( -48.66712064925836501, -0.2684213679329330304, 8.095633725969744177 ) ) ;
#6594=AXIS2_PLACEMENT_3D ( 'NONE', #33765, #48758, #8501 ) ;
#6597=CARTESIAN_POINT ( 'NONE',  ( -12.58062741647496274, -29.25281707778071549, -4.759732266940785550 ) ) ;
#6631=CARTESIAN_POINT ( 'NONE',  ( -13.98431177871173858, -30.12623156650373701, -5.679219063900182718 ) ) ;
#6633=EDGE_CURVE ( 'NONE', #11368, #11657, #43509, .T. ) ;
#6645=DIRECTION ( 'NONE',  ( -1.000000000000000000, 0.000000000000000000, 0.000000000000000000 ) ) ;
#6667=CARTESIAN_POINT ( 'NONE',  ( 19.56743653832046803, -33.00000000000000000, -5.000000000000012434 ) ) ;
#6688=CARTESIAN_POINT ( 'NONE',  ( 47.45484198363494954, -0.5059748548177207539, -8.508429091481751527 ) ) ;
#6716=CARTESIAN_POINT ( 'NONE',  ( 14.33157020395877268, -34.50275931095526261, -8.076358832434346269 ) ) ;
#6718=DIRECTION ( 'NONE',  ( 0.000000000000000000, -1.000000000000000000, 0.000000000000000000 ) ) ;
#6721=CYLINDRICAL_SURFACE ( 'NONE', #6895, 25.00000000000000000 ) ;
#6758=VECTOR ( 'NONE', #49704, 1000.000000000000000 ) ;
#6783=CARTESIAN_POINT ( 'NONE',  ( 1.717027338329501829, -31.08339181399450979, 14.39386062070807171 ) ) ;
#6800=CARTESIAN_POINT ( 'NONE',  ( 0.000000000000000000, -33.00000000000000000, 0.000000000000000000 ) ) ;
#6837=DIRECTION ( 'NONE',  ( 0.000000000000000000, 1.000000000000000000, 0.000000000000000000 ) ) ;
#6873=CARTESIAN_POINT ( 'NONE',  ( -32.70177428389710883, -2.904144763113407191, 22.74422317523286807 ) ) ;
#6878=ORIENTED_EDGE ( 'NONE', *, *, #64874, .F. ) ;
#6895=AXIS2_PLACEMENT_3D ( 'NONE', #21337, #36950, #32603 ) ;
#6898=CARTESIAN_POINT ( 'NONE',  ( 0.000000000000000000, 244.9489742783177917, 156.8996349149244054 ) ) ;
#6920=CARTESIAN_POINT ( 'NONE',  ( -13.50035326695106797, -34.20038524408859359, -9.091202907900893138 ) ) ;
#6951=CARTESIAN_POINT ( 'NONE',  ( -14.30187556442842656, -30.10361765235625597, -4.782130246577440680 ) ) ;
#6954=ORIENTED_EDGE ( 'NONE', *, *, #29375, .F. ) ;
#7021=CARTESIAN_POINT ( 'NONE',  ( 8.240410296153493519, -29.00819526741761578, -11.87861853819113733 ) ) ;
#7028=CARTESIAN_POINT ( 'NONE',  ( 6.824632601691471123, -31.95616727126968115, -13.35541573562854722 ) ) ;
#7030=EDGE_CURVE ( 'NONE', #38363, #33343, #41061, .T. ) ;
#7059=CARTESIAN_POINT ( 'NONE',  ( 18.57729641407469501, -29.86520738451960355, -7.358162954095295305 ) ) ;
#7082=ORIENTED_EDGE ( 'NONE', *, *, #53860, .F. ) ;
#7092=CARTESIAN_POINT ( 'NONE',  ( 4.225235259830817824, -25.92188032005471143, 15.36840686706593928 ) ) ;
#7141=AXIS2_PLACEMENT_3D ( 'NONE', #29736, #24427, #60334 ) ;
#7159=DIRECTION ( 'NONE',  ( 0.9688695217174486674, 0.000000000000000000, 0.2475719085175097645 ) ) ;
#7171=CARTESIAN_POINT ( 'NONE',  ( -14.43403921783542287, -30.05772736395422484, 4.235651140255900060 ) ) ;
#7174=CARTESIAN_POINT ( 'NONE',  ( -31.24126863879125438, -3.096129103239070091, -23.22707964006411530 ) ) ;
#7205=EDGE_LOOP ( 'NONE', ( #28347, #58719, #31948, #35863 ) ) ;
#7210=EDGE_LOOP ( 'NONE', ( #38580, #44876 ) ) ;
#7221=CARTESIAN_POINT ( 'NONE',  ( -16.02805653289875920, -28.24868299250882941, -10.29995797863329621 ) ) ;
#7246=MANIFOLD_SOLID_BREP ( 'Move Face1', #25976 ) ;
#7254=CARTESIAN_POINT ( 'NONE',  ( -19.56743653832047158, -30.00000000000000355, -5.000000000000000888 ) ) ;
#7284=CARTESIAN_POINT ( 'NONE',  ( 19.56743653832047158, -30.00000000000000000, -5.000000000000000888 ) ) ;
#7299=AXIS2_PLACEMENT_3D ( 'NONE', #36236, #45564, #35590 ) ;
#7304=CARTESIAN_POINT ( 'NONE',  ( -1.846890694235063357, -30.59587057577333624, 15.23951446459229864 ) ) ;
#7305=EDGE_CURVE ( 'NONE', #18880, #939, #45455, .T. ) ;
#7333=VERTEX_POINT ( 'NONE', #22943 ) ;
#7340=CARTESIAN_POINT ( 'NONE',  ( 10.63582125256380806, -33.14335888457106449, -11.52436878476450133 ) ) ;
#7391=DIRECTION ( 'NONE',  ( -1.000000000000000000, 0.000000000000000000, 0.000000000000000000 ) ) ;
#7411=ORIENTED_EDGE ( 'NONE', *, *, #57736, .T. ) ;
#7467=DIRECTION ( 'NONE',  ( 0.000000000000000000, 0.000000000000000000, -1.000000000000000000 ) ) ;
#7484=FACE_OUTER_BOUND ( 'NONE', #1323, .T. ) ;
#7500=CARTESIAN_POINT ( 'NONE',  ( -30.43939922888039007, -3.192189569316896236, 23.38849890424057065 ) ) ;
#7504=VECTOR ( 'NONE', #31319, 1000.000000000000000 ) ;
#7553=DIRECTION ( 'NONE',  ( 0.000000000000000000, 0.000000000000000000, -1.000000000000000000 ) ) ;
#7566=AXIS2_PLACEMENT_3D ( 'NONE', #32129, #62383, #51476 ) ;
#7587=ORIENTED_EDGE ( 'NONE', *, *, #40675, .T. ) ;
#7601=ORIENTED_EDGE ( 'NONE', *, *, #20965, .T. ) ;
#7633=CIRCLE ( 'NONE', #6594, 1.500000000000000222 ) ;
#7653=CARTESIAN_POINT ( 'NONE',  ( 4.308196110052892319E-12, -30.53649492335491189, 15.30974548841782656 ) ) ;
#7679=LINE ( 'NONE', #27964, #8854 ) ;
#7690=CARTESIAN_POINT ( 'NONE',  ( 4.340384785879546570, -31.41030204081753752, -14.02840248442898208 ) ) ;
#7725=CARTESIAN_POINT ( 'NONE',  ( 5.029029651858271777, -26.84634345473923034, -15.78007771861069486 ) ) ;
#7763=CARTESIAN_POINT ( 'NONE',  ( 12.80904563207495350, -29.07871018746164538, 3.648338481107272546 ) ) ;
#7786=CIRCLE ( 'NONE', #37484, 22.50555349946515449 ) ;
#7792=EDGE_CURVE ( 'NONE', #17827, #41367, #28802, .T. ) ;
#7815=CARTESIAN_POINT ( 'NONE',  ( 0.8745425597690195119, -31.03649492335506110, 14.44372008463322921 ) ) ;
#7836=CARTESIAN_POINT ( 'NONE',  ( -37.25000000000000711, -1.694065894508600678E-18, 1.500000000000000222 ) ) ;
#7841=DIRECTION ( 'NONE',  ( 0.000000000000000000, 1.000000000000000000, 0.000000000000000000 ) ) ;
#7852=SHAPE_DEFINITION_REPRESENTATION ( #39172, #29683 ) ;
#7854=CARTESIAN_POINT ( 'NONE',  ( -11.31614860309221626, -29.68432482266610606, 9.654990830002102342 ) ) ;
#7858=CARTESIAN_POINT ( 'NONE',  ( -26.58564210842043707, -3.638521970294202657, 24.00000000000000355 ) ) ;
#7869=DIRECTION ( 'NONE',  ( 0.000000000000000000, 1.000000000000000000, 0.000000000000000000 ) ) ;
#7894=EDGE_CURVE ( 'NONE', #16757, #53403, #37391, .T. ) ;
#7915=AXIS2_PLACEMENT_3D ( 'NONE', #41141, #61424, #1266 ) ;
#7938=CARTESIAN_POINT ( 'NONE',  ( -41.00000000000000711, -25.03188948156373073, -4.500000000000008882 ) ) ;
#8017=ORIENTED_EDGE ( 'NONE', *, *, #21381, .T. ) ;
#8031=CARTESIAN_POINT ( 'NONE',  ( 8.395146353820784668, -32.40713589851601739, -12.72020452408354529 ) ) ;
#8057=EDGE_CURVE ( 'NONE', #65704, #44894, #4128, .T. ) ;
#8062=CARTESIAN_POINT ( 'NONE',  ( 17.13446681924518700, -29.51054447109571299, -9.416006455614729376 ) ) ;
#8075=ORIENTED_EDGE ( 'NONE', *, *, #54374, .T. ) ;
#8076=CARTESIAN_POINT ( 'NONE',  ( 37.25000000000000711, -27.21021009056489248, -4.500000000000000888 ) ) ;
#8092=CARTESIAN_POINT ( 'NONE',  ( 13.20768530587737288, -34.09315906254132500, 9.434917751661075158 ) ) ;
#8106=DIRECTION ( 'NONE',  ( 0.000000000000000000, 0.000000000000000000, 1.000000000000000000 ) ) ;
#8147=VERTEX_POINT ( 'NONE', #16705 ) ;
#8159=CARTESIAN_POINT ( 'NONE',  ( 41.00000000000000711, -1.694065894508600678E-18, 0.000000000000000000 ) ) ;
#8167=CARTESIAN_POINT ( 'NONE',  ( -0.8948477690461620337, -30.54755392045577622, 15.29677453898827721 ) ) ;
#8186=CARTESIAN_POINT ( 'NONE',  ( -37.25000000000000711, -27.21021009056489603, 4.499999999999997335 ) ) ;
#8214=DIRECTION ( 'NONE',  ( 0.000000000000000000, 0.000000000000000000, 1.000000000000000000 ) ) ;
#8220=CARTESIAN_POINT ( 'NONE',  ( -10.55354650058127319, -33.11426855636985778, -11.57717840647777408 ) ) ;
#8262=DIRECTION ( 'NONE',  ( -0.9688695217174486674, 0.000000000000000000, 0.2475719085175094036 ) ) ;
#8280=EDGE_CURVE ( 'NONE', #2269, #11657, #10809, .T. ) ;
#8294=DIRECTION ( 'NONE',  ( 0.000000000000000000, 0.000000000000000000, -1.000000000000000000 ) ) ;
#8305=CARTESIAN_POINT ( 'NONE',  ( -7.613843340936869097, -31.56230424472492757, 13.96789312046862896 ) ) ;
#8327=AXIS2_PLACEMENT_3D ( 'NONE', #18500, #64649, #12807 ) ;
#8333=AXIS2_PLACEMENT_3D ( 'NONE', #45899, #9991, #9638 ) ;
#8357=VERTEX_POINT ( 'NONE', #20281 ) ;
#8360=CARTESIAN_POINT ( 'NONE',  ( -25.00000000000000355, -9.999999999999998224, 5.000000000000000888 ) ) ;
#8404=CARTESIAN_POINT ( 'NONE',  ( -22.00000000000000711, -20.00000000000000000, -1.499999999999998002 ) ) ;
#8406=CARTESIAN_POINT ( 'NONE',  ( 19.27363075669222425, -28.98570064806743929, 5.846556568011616939 ) ) ;
#8437=ADVANCED_FACE ( 'NONE', ( #2310, #22242, #16932 ), #41873, .F. ) ;
#8486=CARTESIAN_POINT ( 'NONE',  ( -6.246056400524789609, -31.23659747722503610, 14.42616998329125089 ) ) ;
#8490=CARTESIAN_POINT ( 'NONE',  ( -41.00000000000000711, -1.694065894508793271E-18, 4.500000000000001776 ) ) ;
#8494=CARTESIAN_POINT ( 'NONE',  ( -25.00000000000000355, -30.00000000000000000, 1.530808498934191521E-15 ) ) ;
#8501=DIRECTION ( 'NONE',  ( 0.000000000000000000, 0.000000000000000000, 1.000000000000000000 ) ) ;
#8505=DIRECTION ( 'NONE',  ( 1.000000000000000000, 0.000000000000000000, 0.000000000000000000 ) ) ;
#8537=CARTESIAN_POINT ( 'NONE',  ( -6.778443870680312067, -26.22850392868687663, -14.88193859458597856 ) ) ;
#8575=FACE_OUTER_BOUND ( 'NONE', #7210, .T. ) ;
#8603=CARTESIAN_POINT ( 'NONE',  ( 41.00000000000000711, -25.03188948156373428, -4.500000000000011546 ) ) ;
#8629=CARTESIAN_POINT ( 'NONE',  ( -11.19906371800731471, -32.63487729457052922, 12.17775756912622676 ) ) ;
#8708=TOROIDAL_SURFACE ( 'NONE', #42656, 20.19615242270663558, 3.000000000000000000 ) ;
#8717=DIRECTION ( 'NONE',  ( 0.000000000000000000, 0.000000000000000000, 1.000000000000000000 ) ) ;
#8726=CARTESIAN_POINT ( 'NONE',  ( 40.42380607987477958, -25.46069350086628091, -4.500000000000000888 ) ) ;
#8807=ORIENTED_EDGE ( 'NONE', *, *, #36821, .T. ) ;
#8826=CARTESIAN_POINT ( 'NONE',  ( -1.825668173474303435, -28.16298946971622996, 13.82820292525738459 ) ) ;
#8854=VECTOR ( 'NONE', #48272, 1000.000000000000000 ) ;
#8875=CARTESIAN_POINT ( 'NONE',  ( 5.926183177043330197, -31.73296902231061978, -13.63811545878544607 ) ) ;
#8943=DIRECTION ( 'NONE',  ( 0.000000000000000000, 0.000000000000000000, 1.000000000000000000 ) ) ;
#8953=CARTESIAN_POINT ( 'NONE',  ( 15.59244419633001222, -34.16973227397326696, -7.752328951098071741 ) ) ;
#8987=DIRECTION ( 'NONE',  ( 0.000000000000000000, 0.000000000000000000, 1.000000000000000000 ) ) ;
#8998=CARTESIAN_POINT ( 'NONE',  ( -0.4601472316530035300, -30.53649492335513926, -15.30974548841756189 ) ) ;
#9020=DIRECTION ( 'NONE',  ( -1.000000000000000000, 0.000000000000000000, -0.000000000000000000 ) ) ;
#9022=CARTESIAN_POINT ( 'NONE',  ( 2.022082860508907398, -26.59007814299271288, 16.17076096363556204 ) ) ;
#9032=EDGE_CURVE ( 'NONE', #41515, #16757, #59575, .T. ) ;
#9060=CARTESIAN_POINT ( 'NONE',  ( -8.639472567035785033, -29.08579227083643559, -11.67554154369979358 ) ) ;
#9128=CARTESIAN_POINT ( 'NONE',  ( 25.00000000000000355, -30.00000000000000000, 25.00000000000000000 ) ) ;
#9140=CARTESIAN_POINT ( 'NONE',  ( 3.194234995343356420, -28.25772741626087736, 13.63608895903861118 ) ) ;
#9186=CARTESIAN_POINT ( 'NONE',  ( -8.315422948566315142, -32.37591480791618892, -12.77210737139424523 ) ) ;
#9195=DIRECTION ( 'NONE',  ( -1.000000000000000000, -0.000000000000000000, -0.000000000000000000 ) ) ;
#9225=EDGE_CURVE ( 'NONE', #11368, #34549, #56381, .T. ) ;
#9228=FACE_OUTER_BOUND ( 'NONE', #51913, .T. ) ;
#9242=VERTEX_POINT ( 'NONE', #52029 ) ;
#9254=CARTESIAN_POINT ( 'NONE',  ( 10.04668509498159601, -32.26295471731898346, -12.85148783289987939 ) ) ;
#9299=ORIENTED_EDGE ( 'NONE', *, *, #21661, .F. ) ;
#9301=CARTESIAN_POINT ( 'NONE',  ( -16.48166895389446296, -34.42998396492354374, -6.120168360281142306 ) ) ;
#9318=AXIS2_PLACEMENT_3D ( 'NONE', #32033, #61639, #56691 ) ;
#9321=DIRECTION ( 'NONE',  ( 0.000000000000000000, 0.000000000000000000, -1.000000000000000000 ) ) ;
#9323=CARTESIAN_POINT ( 'NONE',  ( -18.06522620542768820, -29.74877956674518487, 8.189528952361769143 ) ) ;
#9365=CARTESIAN_POINT ( 'NONE',  ( 4.225235259830945722, -26.75987402110986579, -15.91411249164890407 ) ) ;
#9370=ORIENTED_EDGE ( 'NONE', *, *, #11023, .F. ) ;
#9373=CYLINDRICAL_SURFACE ( 'NONE', #53923, 1.500000000000000222 ) ;
#9408=CARTESIAN_POINT ( 'NONE',  ( -47.41971561978370175, -0.5128904950766028925, -11.09198065024577851 ) ) ;
#9440=CARTESIAN_POINT ( 'NONE',  ( -9.081998980629425233, -32.61802400030150295, 12.41144404786857081 ) ) ;
#9453=CARTESIAN_POINT ( 'NONE',  ( 15.07617326819577741, -33.99933334076661851, 8.515830899730941539 ) ) ;
#9485=CARTESIAN_POINT ( 'NONE',  ( -37.25000000000000711, -45.00200000000000244, -4.500000000000000888 ) ) ;
#9500=CARTESIAN_POINT ( 'NONE',  ( -0.8584944786142326700, -27.82166925786467004, -12.56635396443958719 ) ) ;
#9516=CIRCLE ( 'NONE', #38200, 1.500000000000000222 ) ;
#9544=CARTESIAN_POINT ( 'NONE',  ( 17.05023968204110929, -34.50000000000000000, 4.356789313881321846 ) ) ;
#9557=VECTOR ( 'NONE', #40743, 1000.000000000000000 ) ;
#9559=CIRCLE ( 'NONE', #64810, 250.0000000000000000 ) ;
#9562=ORIENTED_EDGE ( 'NONE', *, *, #31291, .T. ) ;
#9567=CARTESIAN_POINT ( 'NONE',  ( 41.00000000000000711, -1.694065894508600678E-18, 1.500000000000000222 ) ) ;
#9573=CARTESIAN_POINT ( 'NONE',  ( 11.20282697758643842, -32.63606470323338726, -12.17568710599035420 ) ) ;
#9581=CARTESIAN_POINT ( 'NONE',  ( -13.93947072118460007, -33.60066931048350369, 9.878030726377206250 ) ) ;
#9617=DIRECTION ( 'NONE',  ( 0.000000000000000000, 0.000000000000000000, 1.000000000000000000 ) ) ;
#9629=CARTESIAN_POINT ( 'NONE',  ( 1.989990211274497156, -25.75944405492161593, 15.61385975544041038 ) ) ;
#9638=DIRECTION ( 'NONE',  ( 0.000000000000000000, 0.000000000000000000, -1.000000000000000000 ) ) ;
#9641=ORIENTED_EDGE ( 'NONE', *, *, #55033, .T. ) ;
#9646=ORIENTED_EDGE ( 'NONE', *, *, #48806, .F. ) ;
#9647=DIRECTION ( 'NONE',  ( 0.000000000000000000, 1.000000000000000000, 0.000000000000000000 ) ) ;
#9665=AXIS2_PLACEMENT_3D ( 'NONE', #19845, #51100, #35763 ) ;
#9667=AXIS2_PLACEMENT_3D ( 'NONE', #3209, #7869, #24131 ) ;
#9701=CARTESIAN_POINT ( 'NONE',  ( -10.20982488791469223, -27.71818678970560867, -14.28592212877975420 ) ) ;
#9749=CARTESIAN_POINT ( 'NONE',  ( 35.31912638668784155, -2.544741887441788197, 22.78557353984778899 ) ) ;
#9782=CARTESIAN_POINT ( 'NONE',  ( -19.56743653832047158, -29.00000000000000000, 5.000000000000000888 ) ) ;
#9792=CARTESIAN_POINT ( 'NONE',  ( 11.89229108778294730, -32.87417574757987637, 11.69979538107606665 ) ) ;
#9843=CARTESIAN_POINT ( 'NONE',  ( 10.20102756488484275, -26.83656875578374112, -13.80782716569073010 ) ) ;
#9872=EDGE_CURVE ( 'NONE', #38736, #38939, #36525, .T. ) ;
#9875=CYLINDRICAL_SURFACE ( 'NONE', #59505, 4.500000000000000888 ) ;
#9922=AXIS2_PLACEMENT_3D ( 'NONE', #25627, #22617, #18629 ) ;
#9981=VERTEX_POINT ( 'NONE', #7284 ) ;
#9984=CARTESIAN_POINT ( 'NONE',  ( 5.446351735594769927, -26.05211744559319342, 15.16580142939698383 ) ) ;
#9991=DIRECTION ( 'NONE',  ( -1.000000000000000000, -0.000000000000000000, -0.000000000000000000 ) ) ;
#10005=CARTESIAN_POINT ( 'NONE',  ( -14.99915657824959325, -28.92607294587372380, 11.47448459775363538 ) ) ;
#10040=CARTESIAN_POINT ( 'NONE',  ( 0.000000000000000000, 0.000000000000000000, 0.000000000000000000 ) ) ;
#10046=CARTESIAN_POINT ( 'NONE',  ( 3.643024398545976261, -28.29981509102550419, -13.54931501599924815 ) ) ;
#10082=CARTESIAN_POINT ( 'NONE',  ( 37.25000000000000711, -1.694065894508600678E-18, 0.000000000000000000 ) ) ;
#10089=CARTESIAN_POINT ( 'NONE',  ( 44.86048679285936913, -0.9948977233718069302, 15.27141897285095951 ) ) ;
#10091=CARTESIAN_POINT ( 'NONE',  ( -49.19530910174992044, -0.1631003452855646629, -6.502801691937063033 ) ) ;
#10095=CARTESIAN_POINT ( 'NONE',  ( 11.20282697759287771, -32.63606470323558284, 12.17568710598608028 ) ) ;
#10116=CARTESIAN_POINT ( 'NONE',  ( -39.82770826892757299, -25.90431001312668968, 4.499999999999997335 ) ) ;
#10120=CARTESIAN_POINT ( 'NONE',  ( -8.775649586809111113, -28.78513225414202026, 9.890132258253697017 ) ) ;
#10131=CARTESIAN_POINT ( 'NONE',  ( 18.66975156949834513, -29.88417193384195159, 7.188590896528484819 ) ) ;
#10165=CARTESIAN_POINT ( 'NONE',  ( 15.96337567072113650, -34.98223374851989576, 4.998641903492888616 ) ) ;
#10173=CARTESIAN_POINT ( 'NONE',  ( 15.45515798858408907, -34.86679772354910511, -6.222782430144768284 ) ) ;
#10186=FACE_BOUND ( 'NONE', #26852, .T. ) ;
#10277=EDGE_LOOP ( 'NONE', ( #28068, #25256, #62941, #16891, #51375, #41468 ) ) ;
#10285=ORIENTED_EDGE ( 'NONE', *, *, #65148, .T. ) ;
#10295=CARTESIAN_POINT ( 'NONE',  ( 13.26780778037857900, -27.53645921949368258, 12.33502842928021792 ) ) ;
#10316=CARTESIAN_POINT ( 'NONE',  ( -15.65911990706704593, -28.15205781829745035, -10.62195165830229726 ) ) ;
#10338=CARTESIAN_POINT ( 'NONE',  ( 45.36026561873625695, -0.9018867892165788325, -12.73108497882287793 ) ) ;
#10355=CARTESIAN_POINT ( 'NONE',  ( -1.806230668642109460, -30.59323697347973336, -15.24264478004127987 ) ) ;
#10432=CARTESIAN_POINT ( 'NONE',  ( -14.82145243739236129, -34.67135967094819193, 7.359580590752245577 ) ) ;
#10435=ORIENTED_EDGE ( 'NONE', *, *, #6633, .T. ) ;
#10442=CARTESIAN_POINT ( 'NONE',  ( 4.513117160428492980, -30.90576903066112990, 14.85933548762089274 ) ) ;
#10490=CARTESIAN_POINT ( 'NONE',  ( 12.85491158824215496, -28.99999999999999645, -3.284771503683511007 ) ) ;
#10491=EDGE_LOOP ( 'NONE', ( #14427, #35217, #39288, #1397 ) ) ;
#10501=ORIENTED_EDGE ( 'NONE', *, *, #45732, .F. ) ;
#10511=ORIENTED_EDGE ( 'NONE', *, *, #43169, .F. ) ;
#10542=DIRECTION ( 'NONE',  ( 0.000000000000000000, 0.000000000000000000, 1.000000000000000000 ) ) ;
#10613=CARTESIAN_POINT ( 'NONE',  ( 16.71517827323052430, -28.42750353049531498, 9.642361815241610401 ) ) ;
#10632=AXIS2_PLACEMENT_3D ( 'NONE', #63737, #58803, #28193 ) ;
#10636=CARTESIAN_POINT ( 'NONE',  ( 9.372867312212076030, -27.54793913079790713, 14.59713702163756288 ) ) ;
#10665=CARTESIAN_POINT ( 'NONE',  ( 35.62380706382416662, -2.504225566391072189, -21.57767586339569732 ) ) ;
#10682=CARTESIAN_POINT ( 'NONE',  ( 13.98043512791030096, -30.12632228061958273, -5.689268883804940558 ) ) ;
#10692=CARTESIAN_POINT ( 'NONE',  ( -6.824045466191706488, -31.96248520358720668, 13.34027024243480319 ) ) ;
#10703=CARTESIAN_POINT ( 'NONE',  ( -25.00000000000000355, -9.999999999999998224, -25.00000000000000000 ) ) ;
#10729=AXIS2_PLACEMENT_3D ( 'NONE', #60754, #49795, #50464 ) ;
#10743=CARTESIAN_POINT ( 'NONE',  ( -37.25000000000000711, -20.00000000000000000, -1.499999999999998002 ) ) ;
#10767=CARTESIAN_POINT ( 'NONE',  ( -12.50548042261300097, -29.27747730776768975, 5.013933227252732827 ) ) ;
#10779=CARTESIAN_POINT ( 'NONE',  ( 13.26995653566893019, -33.36016745060648958, 10.56634385159335388 ) ) ;
#10809=CIRCLE ( 'NONE', #3397, 24.00000000000000000 ) ;
#10831=CARTESIAN_POINT ( 'NONE',  ( 16.03117610287102579, -28.25087052915268870, -10.32844618003480619 ) ) ;
#10833=ADVANCED_FACE ( 'NONE', ( #43947 ), #31400, .F. ) ;
#10840=DIRECTION ( 'NONE',  ( 0.9688695217174486674, 0.000000000000000000, 0.2475719085175097645 ) ) ;
#10927=DIRECTION ( 'NONE',  ( 0.000000000000000000, 0.000000000000000000, 1.000000000000000000 ) ) ;
#10952=CARTESIAN_POINT ( 'NONE',  ( -45.77110135055801265, -0.8256172497425255941, 12.04909734191307003 ) ) ;
#10978=EDGE_CURVE ( 'NONE', #64767, #52558, #39421, .T. ) ;
#10983=AXIS2_PLACEMENT_3D ( 'NONE', #45431, #45769, #54459 ) ;
#10991=CARTESIAN_POINT ( 'NONE',  ( 7.002886717044668252, -27.11012757947471741, 15.35900505431296281 ) ) ;
#11023=EDGE_CURVE ( 'NONE', #57274, #39511, #44112, .T. ) ;
#11027=ORIENTED_EDGE ( 'NONE', *, *, #41730, .F. ) ;
#11031=CARTESIAN_POINT ( 'NONE',  ( 16.79298069408831751, -34.48269025770164120, -5.249417709786706965 ) ) ;
#11056=ORIENTED_EDGE ( 'NONE', *, *, #52253, .T. ) ;
#11059=DIRECTION ( 'NONE',  ( 0.000000000000000000, 1.000000000000000000, 0.000000000000000000 ) ) ;
#11063=CARTESIAN_POINT ( 'NONE',  ( -41.00000000000000711, -1.694065894508793271E-18, 4.500000000000001776 ) ) ;
#11075=CARTESIAN_POINT ( 'NONE',  ( 0.000000000000000000, -33.00000000000000000, 0.000000000000000000 ) ) ;
#11086=ORIENTED_EDGE ( 'NONE', *, *, #48249, .T. ) ;
#11088=DIRECTION ( 'NONE',  ( 0.000000000000000000, 0.000000000000000000, 1.000000000000000000 ) ) ;
#11112=CARTESIAN_POINT ( 'NONE',  ( 15.30590914263659386, -28.05839919878968303, 10.93630420992710128 ) ) ;
#11160=CARTESIAN_POINT ( 'NONE',  ( 0.000000000000000000, -45.00000000000000000, -23.66025403784440684 ) ) ;
#11280=CARTESIAN_POINT ( 'NONE',  ( -16.81745777873098646, -34.49999999816794372, -5.267778333666905510 ) ) ;
#11307=B_SPLINE_CURVE_WITH_KNOTS ( 'NONE', 3,
 ( #17250, #46516, #55264, #36544, #20019, #27219, #56852, #971 ),
 .UNSPECIFIED., .F., .F.,
 ( 4, 2, 2, 4 ),
 ( 0.01146705142166408280, 0.01597709677061664654, 0.01823211944509292928, 0.02048714211956921202 ),
 .UNSPECIFIED. ) ;
#11313=CARTESIAN_POINT ( 'NONE',  ( 4.953976645022760472, -25.99587143922706645, -15.25378271594936841 ) ) ;
#11314=CARTESIAN_POINT ( 'NONE',  ( 18.04777717444646612, -29.74456712077427412, 8.215504029118749330 ) ) ;
#11328=ADVANCED_FACE ( 'NONE', ( #284 ), #16217, .F. ) ;
#11348=CARTESIAN_POINT ( 'NONE',  ( 15.82775651593353672, -34.24354600359633594, -7.361827980272592775 ) ) ;
#11355=CARTESIAN_POINT ( 'NONE',  ( -13.53218314550735357, -34.21215502346591819, 9.055742533985885245 ) ) ;
#11368=VERTEX_POINT ( 'NONE', #17854 ) ;
#11422=CARTESIAN_POINT ( 'NONE',  ( 11.58535936493820273, -27.13779202276463920, 13.20710129366601926 ) ) ;
#11487=AXIS2_PLACEMENT_3D ( 'NONE', #45149, #65408, #19875 ) ;
#11496=CARTESIAN_POINT ( 'NONE',  ( -17.05023968204110929, -34.50000000000000000, 4.356789313881321846 ) ) ;
#11538=AXIS2_PLACEMENT_3D ( 'NONE', #33341, #59850, #4659 ) ;
#11557=CARTESIAN_POINT ( 'NONE',  ( -46.63605190621407814, -0.6629852496305224108, 12.55202432522572664 ) ) ;
#11561=CARTESIAN_POINT ( 'NONE',  ( -15.98984497772178770, -34.99999999818471963, -5.008554314762531767 ) ) ;
#11595=CARTESIAN_POINT ( 'NONE',  ( -19.30028543097103366, -30.00000000000000355, -5.909123879098586052 ) ) ;
#11597=ORIENTED_EDGE ( 'NONE', *, *, #16087, .F. ) ;
#11603=VERTEX_POINT ( 'NONE', #34449 ) ;
#11614=EDGE_CURVE ( 'NONE', #43541, #9242, #54428, .T. ) ;
#11629=CARTESIAN_POINT ( 'NONE',  ( 1.989990211274500043, -25.75944405492161948, -15.61385975544041216 ) ) ;
#11657=VERTEX_POINT ( 'NONE', #26435 ) ;
#11660=CIRCLE ( 'NONE', #57345, 19.00000000000000355 ) ;
#11675=CARTESIAN_POINT ( 'NONE',  ( 11.32672149591984123, -33.39346531321197631, -11.05302976540055582 ) ) ;
#11738=CARTESIAN_POINT ( 'NONE',  ( 7.310206959902322055, -26.30114832292194649, 14.76431686918209785 ) ) ;
#11742=DIRECTION ( 'NONE',  ( -1.000000000000000000, 0.000000000000000000, 0.000000000000000000 ) ) ;
#11760=FACE_OUTER_BOUND ( 'NONE', #10277, .T. ) ;
#11787=CARTESIAN_POINT ( 'NONE',  ( -41.00000000000000711, -25.18551001833413139, 3.766049837354531249 ) ) ;
#11804=CARTESIAN_POINT ( 'NONE',  ( 38.56928140186735021, -26.58605982982061988, -4.500000000000001776 ) ) ;
#11840=CARTESIAN_POINT ( 'NONE',  ( -25.00000000000000355, -30.00000000000000000, 1.530808498934191521E-15 ) ) ;
#11877=ORIENTED_EDGE ( 'NONE', *, *, #28100, .T. ) ;
#11885=CARTESIAN_POINT ( 'NONE',  ( -14.82145243739236129, -34.67135967094819193, -7.359580590752245577 ) ) ;
#11920=CARTESIAN_POINT ( 'NONE',  ( -18.19295774167957092, -29.77901320112238892, -7.993354913176282217 ) ) ;
#11937=DIRECTION ( 'NONE',  ( 1.000000000000000000, -0.000000000000000000, 0.000000000000000000 ) ) ;
#11957=CARTESIAN_POINT ( 'NONE',  ( 18.57729641407471277, -29.86520738451961776, 7.358162954095265107 ) ) ;
#11958=EDGE_CURVE ( 'NONE', #25095, #48019, #7679, .T. ) ;
#12004=DIRECTION ( 'NONE',  ( 0.000000000000000000, 1.000000000000000000, 0.000000000000000000 ) ) ;
#12075=CARTESIAN_POINT ( 'NONE',  ( 11.12775972613914099, -27.03492176219597454, 13.41779706364883396 ) ) ;
#12112=VECTOR ( 'NONE', #41446, 1000.000000000000000 ) ;
#12125=CIRCLE ( 'NONE', #44035, 25.00000000000000000 ) ;
#12136=DIRECTION ( 'NONE',  ( 1.000000000000000000, 0.000000000000000000, 0.000000000000000000 ) ) ;
#12169=CARTESIAN_POINT ( 'NONE',  ( -36.99853283657032677, -2.301590494557429256, 20.84413141647363688 ) ) ;
#12219=CARTESIAN_POINT ( 'NONE',  ( -14.32520573871325631, -34.50054679313745964, -8.085438606780256166 ) ) ;
#12252=CARTESIAN_POINT ( 'NONE',  ( -14.53304282576173279, -30.00000000000001066, -3.713578627762639250 ) ) ;
#12284=CARTESIAN_POINT ( 'NONE',  ( 25.00000000000000355, -30.00000000000000000, 1.530808498934191521E-15 ) ) ;
#12310=ORIENTED_EDGE ( 'NONE', *, *, #889, .F. ) ;
#12334=CARTESIAN_POINT ( 'NONE',  ( 9.537768711902334218, -32.77116127932245604, -12.15562491791137134 ) ) ;
#12444=B_SPLINE_CURVE_WITH_KNOTS ( 'NONE', 3,
 ( #29701, #2839, #35350, #30375, #25067, #30041, #465, #55659, #24739, #40678, #51335, #15407, #10095, #4468, #40332, #40014, #50991, #25717, #45017, #35676, #35003, #773, #50009, #50670, #65292, #61598 ),
 .UNSPECIFIED., .F., .F.,
 ( 4, 2, 2, 2, 2, 2, 2, 2, 2, 2, 2, 2, 4 ),
 ( 0.000000000000000000, 0.001405882151622312804, 0.002811764303244625608, 0.004217646454866938628, 0.005623528606489251215, 0.008435292909733880726, 0.01124705721297850763, 0.01265293936460081849, 0.01405882151622312760, 0.01687058581946774410, 0.01827646797109005322, 0.01968235012271236581, 0.02249411442595698057 ),
 .UNSPECIFIED. ) ;
#12454=CARTESIAN_POINT ( 'NONE',  ( 0.000000000000000000, 244.9489742783177917, -24.99999999999999289 ) ) ;
#12478=CARTESIAN_POINT ( 'NONE',  ( -15.07969093506218883, -34.00054679313987549, 8.511206496389501552 ) ) ;
#12481=CARTESIAN_POINT ( 'NONE',  ( -48.22764741571072022, -0.3553121838687482437, -6.242084797467388313 ) ) ;
#12507=LINE ( 'NONE', #58768, #22354 ) ;
#12521=CARTESIAN_POINT ( 'NONE',  ( -44.83472798829954797, -0.9996270273486108637, 15.30615170800020763 ) ) ;
#12529=CARTESIAN_POINT ( 'NONE',  ( -12.75996857643550797, -29.16082758670667019, -4.038023594093941959 ) ) ;
#12542=CARTESIAN_POINT ( 'NONE',  ( -19.56743653832047158, -33.00000000000000000, -5.000000000000003553 ) ) ;
#12552=ORIENTED_EDGE ( 'NONE', *, *, #27463, .F. ) ;
#12561=CARTESIAN_POINT ( 'NONE',  ( -13.26547918569663054, -33.36007533429795302, -10.54465099870413880 ) ) ;
#12567=ORIENTED_EDGE ( 'NONE', *, *, #53667, .T. ) ;
#12583=CARTESIAN_POINT ( 'NONE',  ( -25.00000000000000355, -30.00000000000000000, 5.000000000000000888 ) ) ;
#12608=CARTESIAN_POINT ( 'NONE',  ( 3.657075258460736222, -30.77912794045597522, -15.01778408663798814 ) ) ;
#12649=CARTESIAN_POINT ( 'NONE',  ( 14.81924285005568898, -34.67057711548255128, -7.362581078982665339 ) ) ;
#12672=ADVANCED_FACE ( 'NONE', ( #55438 ), #9875, .T. ) ;
#12675=ORIENTED_EDGE ( 'NONE', *, *, #48029, .T. ) ;
#12686=CARTESIAN_POINT ( 'NONE',  ( 5.527856869237409931, -26.90719658711817530, -15.68471180892751171 ) ) ;
#12722=CARTESIAN_POINT ( 'NONE',  ( 12.30974346995382973, -29.30943841933768113, 5.552318955347200991 ) ) ;
#12741=VERTEX_POINT ( 'NONE', #38338 ) ;
#12807=DIRECTION ( 'NONE',  ( 0.000000000000000000, 0.000000000000000000, 1.000000000000000000 ) ) ;
#12813=CARTESIAN_POINT ( 'NONE',  ( 4.225235259830817824, -26.75987402111029922, 15.91411249164822728 ) ) ;
#12840=ORIENTED_EDGE ( 'NONE', *, *, #26896, .F. ) ;
#12864=CARTESIAN_POINT ( 'NONE',  ( -36.06592381555557125, -2.436921198044748937, -22.43244911821614807 ) ) ;
#12868=B_SPLINE_CURVE_WITH_KNOTS ( 'NONE', 3,
 ( #8186, #58757, #32456, #43093, #63369, #17837, #37456, #59077 ),
 .UNSPECIFIED., .F., .F.,
 ( 4, 2, 2, 4 ),
 ( 0.01093700429183111326, 0.01319343274642247738, 0.01544986120101383975, 0.01996271811019656450 ),
 .UNSPECIFIED. ) ;
#12875=CARTESIAN_POINT ( 'NONE',  ( -10.50558643126015923, -29.12101583629321766, -8.365681325885642394 ) ) ;
#12922=DIRECTION ( 'NONE',  ( -0.2475719085175105416, 8.403603522408387294E-16, -0.9688695217174485563 ) ) ;
#12929=ORIENTED_EDGE ( 'NONE', *, *, #18267, .T. ) ;
#12932=CARTESIAN_POINT ( 'NONE',  ( 41.00000000000000711, -1.694065894508600678E-18, 1.500000000000000222 ) ) ;
#12945=DIRECTION ( 'NONE',  ( -1.000000000000000000, 0.000000000000000000, 0.000000000000000000 ) ) ;
#12954=CARTESIAN_POINT ( 'NONE',  ( 0.9207726606790023194, -30.53649492335445359, -15.30974548841835592 ) ) ;
#13047=ORIENTED_EDGE ( 'NONE', *, *, #17758, .F. ) ;
#13050=CARTESIAN_POINT ( 'NONE',  ( 41.00000000000000711, 1.820029539775944174E-16, -1.500000000000000222 ) ) ;
#13071=EDGE_CURVE ( 'NONE', #25930, #54896, #3457, .T. ) ;
#13073=CARTESIAN_POINT ( 'NONE',  ( 17.91771366450749525, -28.72671386922736758, 8.232269603669239544 ) ) ;
#13113=CARTESIAN_POINT ( 'NONE',  ( 31.45682506574157244, -3.065323467461853024, -24.16565572891780889 ) ) ;
#13141=DIRECTION ( 'NONE',  ( -1.000000000000000000, 0.000000000000000000, 0.000000000000000000 ) ) ;
#13158=EDGE_CURVE ( 'NONE', #53510, #57274, #32708, .T. ) ;
#13159=CARTESIAN_POINT ( 'NONE',  ( -2.647174210752905488, -26.63290002157760128, 16.10638009382239488 ) ) ;
#13164=DIRECTION ( 'NONE',  ( 1.000000000000000000, -0.000000000000000000, -0.000000000000000000 ) ) ;
#13211=CARTESIAN_POINT ( 'NONE',  ( -2.647174210752905488, -25.80125502049867947, -15.55106108913133767 ) ) ;
#13231=ORIENTED_EDGE ( 'NONE', *, *, #58494, .F. ) ;
#13247=CARTESIAN_POINT ( 'NONE',  ( -19.56743653832047158, -33.00000000000000000, 5.000000000000000888 ) ) ;
#13330=CARTESIAN_POINT ( 'NONE',  ( -19.56743653832047514, -28.99999999999999645, 5.000000000000000888 ) ) ;
#13347=DIRECTION ( 'NONE',  ( -0.000000000000000000, 1.000000000000000000, -0.000000000000000000 ) ) ;
#13369=ORIENTED_EDGE ( 'NONE', *, *, #889, .T. ) ;
#13390=CARTESIAN_POINT ( 'NONE',  ( 12.19204271345157586, -29.31683997938378639, 5.830637565203388384 ) ) ;
#13466=CARTESIAN_POINT ( 'NONE',  ( -9.594501343355146261, -32.11802400029680626, 13.11109426626678953 ) ) ;
#13476=ORIENTED_EDGE ( 'NONE', *, *, #40675, .F. ) ;
#13495=B_SPLINE_CURVE_WITH_KNOTS ( 'NONE', 3,
 ( #55339, #10116, #64327, #44688 ),
 .UNSPECIFIED., .F., .F.,
 ( 4, 4 ),
 ( 0.007620068080905808769, 0.01192914805994312565 ),
 .UNSPECIFIED. ) ;
#13517=CARTESIAN_POINT ( 'NONE',  ( -1.704253825401055966, -31.09323697348121129, -14.38225808330797584 ) ) ;
#13546=EDGE_CURVE ( 'NONE', #64767, #56931, #33052, .T. ) ;
#13605=CARTESIAN_POINT ( 'NONE',  ( -37.25000000000000711, -1.694065894508600678E-18, 0.000000000000000000 ) ) ;
#13665=CARTESIAN_POINT ( 'NONE',  ( -25.00000000000000355, -30.00000000000000000, -24.00000000000000000 ) ) ;
#13707=CARTESIAN_POINT ( 'NONE',  ( 14.05446433506782533, -34.40329588773735736, 8.438602785652603799 ) ) ;
#13731=PLANE ( 'NONE',  #30483 ) ;
#13785=CARTESIAN_POINT ( 'NONE',  ( -4.536586326003440028, -28.39263410566477930, 13.35746355086213555 ) ) ;
#13833=CARTESIAN_POINT ( 'NONE',  ( 4.699914177767785084, -28.11199977926868598, -11.88398404624164506 ) ) ;
#13909=DIRECTION ( 'NONE',  ( 0.000000000000000000, -1.000000000000000000, 0.000000000000000000 ) ) ;
#13924=CARTESIAN_POINT ( 'NONE',  ( -16.48166895389392650, -34.42998396492343716, 6.120168360282491449 ) ) ;
#13955=FACE_OUTER_BOUND ( 'NONE', #56809, .T. ) ;
#13966=AXIS2_PLACEMENT_3D ( 'NONE', #26423, #46704, #1164 ) ;
#13971=CARTESIAN_POINT ( 'NONE',  ( -1.846890694251213771, -30.59587057577444824, -15.23951446459097170 ) ) ;
#13993=ORIENTED_EDGE ( 'NONE', *, *, #9032, .T. ) ;
#14008=CARTESIAN_POINT ( 'NONE',  ( -13.38666790241063964, -28.49056413965659473, -12.64716857254873617 ) ) ;
#14014=EDGE_CURVE ( 'NONE', #61621, #29328, #7633, .T. ) ;
#14037=CARTESIAN_POINT ( 'NONE',  ( -7.454036404616594780, -28.85515183291198227, -12.27947133142141212 ) ) ;
#14095=VERTEX_POINT ( 'NONE', #1159 ) ;
#14123=CARTESIAN_POINT ( 'NONE',  ( -14.91771861688918399, -28.90354855594946315, 11.53870211789912759 ) ) ;
#14175=CARTESIAN_POINT ( 'NONE',  ( 8.295782569430503628, -26.46630966554524278, -14.48708413691750074 ) ) ;
#14207=DIRECTION ( 'NONE',  ( 0.000000000000000000, -0.8660254037844380415, -0.5000000000000009992 ) ) ;
#14213=DIRECTION ( 'NONE',  ( -1.000000000000000000, 0.000000000000000000, 0.000000000000000000 ) ) ;
#14238=AXIS2_PLACEMENT_3D ( 'NONE', #63265, #37996, #1788 ) ;
#14271=CARTESIAN_POINT ( 'NONE',  ( -15.69195845145067736, -33.00000000000000000, -4.009712365929965827 ) ) ;
#14285=PLANE ( 'NONE',  #32110 ) ;
#14351=ADVANCED_FACE ( 'NONE', ( #1000 ), #61835, .F. ) ;
#14367=CARTESIAN_POINT ( 'NONE',  ( 3.194234995343557149, -28.25772741625902640, -13.63608895904094531 ) ) ;
#14374=ORIENTED_EDGE ( 'NONE', *, *, #45732, .T. ) ;
#14405=CARTESIAN_POINT ( 'NONE',  ( 43.79915462856099850, -1.187172983101278056, -16.56021102286108970 ) ) ;
#14427=ORIENTED_EDGE ( 'NONE', *, *, #21982, .T. ) ;
#14435=CARTESIAN_POINT ( 'NONE',  ( -11.25859294448574666, -33.36858074101470351, 11.10377723166772768 ) ) ;
#14443=CARTESIAN_POINT ( 'NONE',  ( -25.00000000000000355, -30.00000000000000000, -24.00000000000000000 ) ) ;
#14444=CARTESIAN_POINT ( 'NONE',  ( 16.45277491483706456, -34.41570230176820644, 6.124363151459176535 ) ) ;
#14446=EDGE_CURVE ( 'NONE', #58655, #30420, #57859, .T. ) ;
#14453=EDGE_LOOP ( 'NONE', ( #34253, #63201, #39961, #53814 ) ) ;
#14466=VERTEX_POINT ( 'NONE', #62477 ) ;
#14491=CARTESIAN_POINT ( 'NONE',  ( 1.717027338329501829, -31.08339181399450979, -14.39386062070807171 ) ) ;
#14513=DIRECTION ( 'NONE',  ( -1.000000000000000000, 0.000000000000000000, -0.000000000000000000 ) ) ;
#14557=ORIENTED_EDGE ( 'NONE', *, *, #57749, .T. ) ;
#14611=CARTESIAN_POINT ( 'NONE',  ( -17.05023968204110929, -34.50000000000000000, -4.356789313881321846 ) ) ;
#14667=DIRECTION ( 'NONE',  ( 1.000000000000000000, 0.000000000000000000, 0.000000000000000000 ) ) ;
#14673=CARTESIAN_POINT ( 'NONE',  ( -13.72965000697286264, -28.58137455677893612, -12.42479717943305140 ) ) ;
#14719=CARTESIAN_POINT ( 'NONE',  ( 47.77550903397572313, -0.4437794964968695410, 10.34167951973068966 ) ) ;
#14728=CIRCLE ( 'NONE', #51941, 5.000000000000000888 ) ;
#14739=ORIENTED_EDGE ( 'NONE', *, *, #23408, .T. ) ;
#14752=CARTESIAN_POINT ( 'NONE',  ( -8.761386526127953545, -26.55543068763903491, 14.32493309394703829 ) ) ;
#14763=CARTESIAN_POINT ( 'NONE',  ( 17.91771366450749525, -29.71233038866033382, 8.402389056494223851 ) ) ;
#14803=CARTESIAN_POINT ( 'NONE',  ( -0.4370662499957438385, -31.03649492335514992, -14.44372008463312795 ) ) ;
#14809=CARTESIAN_POINT ( 'NONE',  ( 10.57252189908326301, -33.12087690403964046, -11.56547414815872088 ) ) ;
#14855=ADVANCED_FACE ( 'NONE', ( #16082 ), #60996, .F. ) ;
#14884=TOROIDAL_SURFACE ( 'NONE', #52088, 20.19615242270663558, 3.000000000000000000 ) ;
#14920=( GEOMETRIC_REPRESENTATION_CONTEXT ( 3 ) GLOBAL_UNCERTAINTY_ASSIGNED_CONTEXT ( ( #17723 ) ) GLOBAL_UNIT_ASSIGNED_CONTEXT ( ( #56197, #20644, #6023 ) ) REPRESENTATION_CONTEXT ( 'NONE', 'WORKASPACE' ) );
#14934=CARTESIAN_POINT ( 'NONE',  ( -22.00000000000000711, -20.00000000000000000, 2.449293598294706907E-15 ) ) ;
#14941=CARTESIAN_POINT ( 'NONE',  ( -2.496508956744591501, -25.79293017570256552, 15.56347233531499086 ) ) ;
#14943=DIRECTION ( 'NONE',  ( 0.000000000000000000, 1.000000000000000000, 0.000000000000000000 ) ) ;
#14945=DIRECTION ( 'NONE',  ( 0.000000000000000000, 0.000000000000000000, -1.000000000000000000 ) ) ;
#14963=ORIENTED_EDGE ( 'NONE', *, *, #63632, .T. ) ;
#14979=FACE_OUTER_BOUND ( 'NONE', #40892, .T. ) ;
#14981=EDGE_CURVE ( 'NONE', #25930, #54875, #62284, .T. ) ;
#15011=CARTESIAN_POINT ( 'NONE',  ( -9.594501343354149725, -32.11802400029404936, -13.11109426626555319 ) ) ;
#15097=CARTESIAN_POINT ( 'NONE',  ( -11.75561129372955094, -29.30098385689712970, 6.671426272442088745 ) ) ;
#15108=CARTESIAN_POINT ( 'NONE',  ( 9.349182579143541005, -29.24123260035452176, 11.20990699596516293 ) ) ;
#15151=CARTESIAN_POINT ( 'NONE',  ( -14.08345347784036328, -34.41374607521908757, -8.401505689976490387 ) ) ;
#15157=CARTESIAN_POINT ( 'NONE',  ( 19.43600575278776788, -28.99999999999999289, -5.424900065531946147 ) ) ;
#15192=VERTEX_POINT ( 'NONE', #8404 ) ;
#15200=ORIENTED_EDGE ( 'NONE', *, *, #55033, .F. ) ;
#15267=CIRCLE ( 'NONE', #52461, 20.19615242270663558 ) ;
#15292=CARTESIAN_POINT ( 'NONE',  ( -12.41459945261391340, -27.32694502519497703, 12.80960016232523024 ) ) ;
#15315=CARTESIAN_POINT ( 'NONE',  ( -6.902482536246134615, -26.23992191484883918, -14.86511077371810963 ) ) ;
#15316=CARTESIAN_POINT ( 'NONE',  ( -6.997870572558772650, -27.10943569200530590, 15.36011607788394784 ) ) ;
#15352=DIRECTION ( 'NONE',  ( 0.000000000000000000, 0.000000000000000000, 1.000000000000000000 ) ) ;
#15355=VERTEX_POINT ( 'NONE', #12583 ) ;
#15357=CARTESIAN_POINT ( 'NONE',  ( 6.263846918920576989, -28.63916073140924112, -12.80708683763842082 ) ) ;
#15365=CARTESIAN_POINT ( 'NONE',  ( 4.037157412408303976E-12, -31.03649492335491544, 14.44372008463339085 ) ) ;
#15400=CARTESIAN_POINT ( 'NONE',  ( 33.05588761701184808, -2.860689001541081744, 23.72276540370177145 ) ) ;
#15407=CARTESIAN_POINT ( 'NONE',  ( 11.92950489381524370, -32.88714273283334677, 11.67197772323657112 ) ) ;
#15422=ORIENTED_EDGE ( 'NONE', *, *, #21982, .F. ) ;
#15427=CARTESIAN_POINT ( 'NONE',  ( 0.000000000000000000, -30.00000000000000000, 0.000000000000000000 ) ) ;
#15431=CARTESIAN_POINT ( 'NONE',  ( -7.278994278378053018, -26.30414574191657096, 14.75709246356266036 ) ) ;
#15441=CARTESIAN_POINT ( 'NONE',  ( 8.240410296153402925, -29.00819526741667076, 11.87861853819304514 ) ) ;
#15443=AXIS2_PLACEMENT_3D ( 'NONE', #6667, #46557, #5694 ) ;
#15566=CARTESIAN_POINT ( 'NONE',  ( 0.000000000000000000, -33.00000000000000000, 0.000000000000000000 ) ) ;
#15592=CARTESIAN_POINT ( 'NONE',  ( -18.91767133624980701, -29.93867241416544545, 6.768471019338283767 ) ) ;
#15609=CARTESIAN_POINT ( 'NONE',  ( 14.88292245651501844, -27.94758995389112854, 11.26211297105860787 ) ) ;
#15615=ORIENTED_EDGE ( 'NONE', *, *, #49745, .F. ) ;
#15647=CARTESIAN_POINT ( 'NONE',  ( 31.19808003874557301, -3.097905286366202660, -23.19915556217947739 ) ) ;
#15648=CARTESIAN_POINT ( 'NONE',  ( 22.00000000000000711, -20.00000000000000000, 1.500000000000002887 ) ) ;
#15662=CARTESIAN_POINT ( 'NONE',  ( 13.74768401152559250, -28.58623978001741861, -12.41178146356746836 ) ) ;
#15692=ADVANCED_FACE ( 'NONE', ( #59007 ), #34414, .F. ) ;
#15742=CARTESIAN_POINT ( 'NONE',  ( -12.81094353615569048, -29.07674955874489342, 3.635823793965939466 ) ) ;
#15744=CARTESIAN_POINT ( 'NONE',  ( 16.66082797316812503, -33.00000000000000000, 4.257284274447473926 ) ) ;
#15753=CARTESIAN_POINT ( 'NONE',  ( 19.56743653832047869, -29.99999999999999645, 4.999999999999984013 ) ) ;
#15782=AXIS2_PLACEMENT_3D ( 'NONE', #13665, #9321, #9020 ) ;
#15795=AXIS2_PLACEMENT_3D ( 'NONE', #4465, #53777, #8214 ) ;
#15843=DIRECTION ( 'NONE',  ( 0.000000000000000000, 0.000000000000000000, -1.000000000000000000 ) ) ;
#15878=VECTOR ( 'NONE', #28718, 1000.000000000000000 ) ;
#15916=CARTESIAN_POINT ( 'NONE',  ( -37.00843563923471891, -2.297594674915165225, -20.79457751400812171 ) ) ;
#15927=CARTESIAN_POINT ( 'NONE',  ( -6.902482536246133726, -26.23992191484884273, 14.86511077371810430 ) ) ;
#15946=ORIENTED_EDGE ( 'NONE', *, *, #29375, .T. ) ;
#15974=CARTESIAN_POINT ( 'NONE',  ( 45.37278721346743282, -0.8995687559120728594, 12.71067884230445344 ) ) ;
#15995=CARTESIAN_POINT ( 'NONE',  ( 15.59065549519859317, -34.16917994668161640, -7.755393724196137484 ) ) ;
#16044=CIRCLE ( 'NONE', #53237, 20.00000000000000000 ) ;
#16082=FACE_OUTER_BOUND ( 'NONE', #45940, .T. ) ;
#16083=CARTESIAN_POINT ( 'NONE',  ( 8.295782569430503628, -26.46630966554524278, 14.48708413691750074 ) ) ;
#16087=EDGE_CURVE ( 'NONE', #31565, #7333, #32309, .T. ) ;
#16094=AXIS2_PLACEMENT_3D ( 'NONE', #27456, #58392, #43401 ) ;
#16170=ORIENTED_EDGE ( 'NONE', *, *, #44360, .T. ) ;
#16196=FACE_OUTER_BOUND ( 'NONE', #40739, .T. ) ;
#16199=ADVANCED_FACE ( 'NONE', ( #53924 ), #42950, .F. ) ;
#16217=CYLINDRICAL_SURFACE ( 'NONE', #7915, 1.500000000000000222 ) ;
#16221=ADVANCED_FACE ( 'NONE', ( #55217 ), #39264, .F. ) ;
#16254=ORIENTED_EDGE ( 'NONE', *, *, #57829, .T. ) ;
#16279=CARTESIAN_POINT ( 'NONE',  ( -15.65911990706704593, -28.15205781829744680, 10.62195165830229726 ) ) ;
#16310=CARTESIAN_POINT ( 'NONE',  ( 10.75388052849570109, -27.84561629232752722, 14.03224735226134712 ) ) ;
#16333=CARTESIAN_POINT ( 'NONE',  ( 46.52334308975179056, -0.6843348755673265282, 10.64746346056991833 ) ) ;
#16347=CARTESIAN_POINT ( 'NONE',  ( 37.25000000000000711, -27.44817602132957646, -3.024649682742619472 ) ) ;
#16351=CARTESIAN_POINT ( 'NONE',  ( 17.02556425888772296, -29.48112685930881227, -9.540979227922154138 ) ) ;
#16355=ORIENTED_EDGE ( 'NONE', *, *, #52243, .F. ) ;
#16359=CARTESIAN_POINT ( 'NONE',  ( -12.31625042011401838, -33.75886355119370563, 10.24605909438714946 ) ) ;
#16374=CIRCLE ( 'NONE', #40759, 5.000000000000000888 ) ;
#16386=CARTESIAN_POINT ( 'NONE',  ( -37.00000000000000711, -45.00200000000000244, -4.500000000000000888 ) ) ;
#16432=CARTESIAN_POINT ( 'NONE',  ( 4.261270162784661863, -31.40576903066106240, 14.03034928007075344 ) ) ;
#16478=ORIENTED_EDGE ( 'NONE', *, *, #28667, .T. ) ;
#16482=CARTESIAN_POINT ( 'NONE',  ( 14.81924285005721131, -34.67057711548305576, 7.362581078980241500 ) ) ;
#16496=CARTESIAN_POINT ( 'NONE',  ( 19.56743653832047158, -33.00000000000000000, 5.000000000000007994 ) ) ;
#16572=DIRECTION ( 'NONE',  ( 0.000000000000000000, 0.000000000000000000, 1.000000000000000000 ) ) ;
#16580=CARTESIAN_POINT ( 'NONE',  ( -25.00000000000000355, -30.00000000000000000, 24.00000000000000000 ) ) ;
#16604=VERTEX_POINT ( 'NONE', #8603 ) ;
#16630=EDGE_LOOP ( 'NONE', ( #25428, #24248, #25587, #13993 ) ) ;
#16631=DIRECTION ( 'NONE',  ( 0.000000000000000000, 1.000000000000000000, 0.000000000000000000 ) ) ;
#16632=CARTESIAN_POINT ( 'NONE',  ( -2.496508956744591057, -25.79293017570256552, -15.56347233531499441 ) ) ;
#16640=CARTESIAN_POINT ( 'NONE',  ( 8.843349564587759559, -31.89871022336092921, -13.45657735392536480 ) ) ;
#16651=CARTESIAN_POINT ( 'NONE',  ( 39.62372872010316627, -1.894461972532903271, 19.09391518418254208 ) ) ;
#16666=CARTESIAN_POINT ( 'NONE',  ( 14.53304282576173634, -29.99999999999999289, -3.713578627762628592 ) ) ;
#16705=CARTESIAN_POINT ( 'NONE',  ( -25.00000000000000355, -3.797884998337192286, -23.99999999999999289 ) ) ;
#16721=ORIENTED_EDGE ( 'NONE', *, *, #59149, .F. ) ;
#16740=CARTESIAN_POINT ( 'NONE',  ( -1.729917593620911020, -27.85289612474432275, 12.49635169356267106 ) ) ;
#16757=VERTEX_POINT ( 'NONE', #46796 ) ;
#16802=CARTESIAN_POINT ( 'NONE',  ( 4.037157412408303976E-12, -31.03649492335491544, 14.44372008463339085 ) ) ;
#16876=CARTESIAN_POINT ( 'NONE',  ( -26.65194590272819042, -3.631858188236755769, 25.00000000000000000 ) ) ;
#16891=ORIENTED_EDGE ( 'NONE', *, *, #45001, .F. ) ;
#16932=FACE_BOUND ( 'NONE', #57881, .T. ) ;
#16960=CARTESIAN_POINT ( 'NONE',  ( -1.318817192132426526E-11, -30.53649492335491544, -15.30974548841782834 ) ) ;
#16998=CARTESIAN_POINT ( 'NONE',  ( 0.000000000000000000, -45.00000000000000000, 0.000000000000000000 ) ) ;
#17065=CARTESIAN_POINT ( 'NONE',  ( 8.088853370213684002, -28.65367229866794219, 10.33367282332777393 ) ) ;
#17125=AXIS2_PLACEMENT_3D ( 'NONE', #34751, #55054, #48779 ) ;
#17143=CARTESIAN_POINT ( 'NONE',  ( -37.25000000000000711, -20.00000000000000000, 1.500000000000002887 ) ) ;
#17162=CARTESIAN_POINT ( 'NONE',  ( -48.79774903324594248, -0.2423453535664360781, -3.134413741627059213 ) ) ;
#17250=CARTESIAN_POINT ( 'NONE',  ( 41.00000000000000711, -25.03188948156373428, -4.500000000000011546 ) ) ;
#17254=CARTESIAN_POINT ( 'NONE',  ( -17.03240540343445986, -29.48295256022982969, -9.532950799340856207 ) ) ;
#17256=ORIENTED_EDGE ( 'NONE', *, *, #40682, .T. ) ;
#17265=ORIENTED_EDGE ( 'NONE', *, *, #35342, .T. ) ;
#17314=CARTESIAN_POINT ( 'NONE',  ( 35.62304844322793684, -2.500997609376311548, 21.53526926371174000 ) ) ;
#17411=CARTESIAN_POINT ( 'NONE',  ( -3.416103270178013407, -31.26314776370590209, 14.19449313401761081 ) ) ;
#17482=PLANE ( 'NONE',  #37871 ) ;
#17497=PRODUCT_CONTEXT ( 'NONE', #27271, 'mechanical' ) ;
#17503=CARTESIAN_POINT ( 'NONE',  ( -37.67868074218839780, -2.196220884325941203, -20.39261666198438760 ) ) ;
#17518=DIRECTION ( 'NONE',  ( 6.123233995736778362E-17, -0.8660254037844380415, 0.5000000000000009992 ) ) ;
#17546=CARTESIAN_POINT ( 'NONE',  ( -47.76247274761328754, -0.4463159248369971688, 10.36992351718251371 ) ) ;
#17561=CARTESIAN_POINT ( 'NONE',  ( 25.00000000000000355, -30.00000000000000000, -5.000000000000000888 ) ) ;
#17563=ORIENTED_EDGE ( 'NONE', *, *, #43993, .F. ) ;
#17577=EDGE_CURVE ( 'NONE', #8147, #33520, #62986, .T. ) ;
#17588=DIRECTION ( 'NONE',  ( -0.9688695217174486674, 0.000000000000000000, 0.2475719085175094036 ) ) ;
#17596=CARTESIAN_POINT ( 'NONE',  ( 25.00000000000000355, -9.999999999999998224, 25.00000000000000000 ) ) ;
#17626=CARTESIAN_POINT ( 'NONE',  ( -18.01523681890432371, -28.74990419755712878, -8.100995087731224231 ) ) ;
#17665=DIRECTION ( 'NONE',  ( 0.2475719085175094591, 0.000000000000000000, -0.9688695217174487784 ) ) ;
#17699=FACE_OUTER_BOUND ( 'NONE', #30389, .T. ) ;
#17709=CARTESIAN_POINT ( 'NONE',  ( 17.75832895199376793, -29.67262258703657807, -8.626345146652873552 ) ) ;
#17713=DIRECTION ( 'NONE',  ( 0.000000000000000000, 0.000000000000000000, 1.000000000000000000 ) ) ;
#17723=UNCERTAINTY_MEASURE_WITH_UNIT (LENGTH_MEASURE( 1.000000000000000082E-05 ), #56197, 'distance_accuracy_value', 'NONE');
#17727=LINE ( 'NONE', #37984, #57219 ) ;
#17758=EDGE_CURVE ( 'NONE', #34549, #939, #44193, .T. ) ;
#17808=DIRECTION ( 'NONE',  ( 0.000000000000000000, 0.000000000000000000, 1.000000000000000000 ) ) ;
#17821=CARTESIAN_POINT ( 'NONE',  ( -44.06649112733600759, -1.138262461040779439, -14.66001971352459243 ) ) ;
#17827=VERTEX_POINT ( 'NONE', #35818 ) ;
#17837=CARTESIAN_POINT ( 'NONE',  ( -37.25000000000002132, -27.56175630915211272, -1.528111002209142422 ) ) ;
#17854=CARTESIAN_POINT ( 'NONE',  ( -25.00000000000000355, -28.99999999999999645, 5.000000000000000888 ) ) ;
#17945=ORIENTED_EDGE ( 'NONE', *, *, #44501, .F. ) ;
#17982=CARTESIAN_POINT ( 'NONE',  ( -19.56743653832047514, -33.00000000000000000, -5.000000000000001776 ) ) ;
#17991=CARTESIAN_POINT ( 'NONE',  ( 9.160076034422203861, -32.64719971958299283, -12.35384511440537381 ) ) ;
#18032=CARTESIAN_POINT ( 'NONE',  ( -37.25000000000000711, -1.694065894508600678E-18, 0.000000000000000000 ) ) ;
#18064=CARTESIAN_POINT ( 'NONE',  ( 12.57831868240780082, -29.25370879966822812, 4.768001503383645812 ) ) ;
#18093=STYLED_ITEM ( 'NONE', ( #61847 ), #7246 ) ;
#18149=CARTESIAN_POINT ( 'NONE',  ( -0.9057367950588101069, -28.12814853318038644, 13.89764383195466912 ) ) ;
#18153=CARTESIAN_POINT ( 'NONE',  ( -47.77118093457291081, -0.4451837999798801682, -7.743266003128062458 ) ) ;
#18167=CARTESIAN_POINT ( 'NONE',  ( 25.00000000000000355, -30.00000000000000000, -25.00000000000000000 ) ) ;
#18207=CARTESIAN_POINT ( 'NONE',  ( -2.136460567204509164, -31.12783502484143128, -14.34456412933875846 ) ) ;
#18258=CARTESIAN_POINT ( 'NONE',  ( -25.00000000000000355, -9.999999999999998224, 1.530808498934191521E-15 ) ) ;
#18262=VERTEX_POINT ( 'NONE', #11160 ) ;
#18267=EDGE_CURVE ( 'NONE', #43036, #25930, #58324, .T. ) ;
#18269=EDGE_CURVE ( 'NONE', #59550, #50924, #2158, .T. ) ;
#18319=VERTEX_POINT ( 'NONE', #42054 ) ;
#18331=CARTESIAN_POINT ( 'NONE',  ( 19.56743653832047514, -30.00000000000000000, 5.000000000000000888 ) ) ;
#18339=CARTESIAN_POINT ( 'NONE',  ( -4.578562111161573078, -30.90741127680607292, -14.86059354493461448 ) ) ;
#18378=VECTOR ( 'NONE', #37248, 1000.000000000000000 ) ;
#18391=CARTESIAN_POINT ( 'NONE',  ( 37.91369172636191820, -26.91879662985438415, -4.500000000000000888 ) ) ;
#18410=CARTESIAN_POINT ( 'NONE',  ( 12.83306155034139096, -29.03814089300163914, 3.459227852998686625 ) ) ;
#18500=CARTESIAN_POINT ( 'NONE',  ( -41.00000000000000711, -1.694065894508600678E-18, 0.000000000000000000 ) ) ;
#18505=CARTESIAN_POINT ( 'NONE',  ( -5.261125060311115931, -26.86576352283317703, 15.75274798952654187 ) ) ;
#18532=AXIS2_PLACEMENT_3D ( 'NONE', #23871, #9195, #23532 ) ;
#18557=CARTESIAN_POINT ( 'NONE',  ( 4.286683309450310730, -28.06227586351231196, -12.00609810331033067 ) ) ;
#18573=CARTESIAN_POINT ( 'NONE',  ( 15.69195845145067381, -33.00000000000000000, -4.009712365929972044 ) ) ;
#18629=DIRECTION ( 'NONE',  ( -1.000000000000000000, 0.000000000000000000, 0.000000000000000000 ) ) ;
#18669=PRODUCT_DEFINITION_FORMATION_WITH_SPECIFIED_SOURCE ( 'ANY', '', #49305, .NOT_KNOWN. ) ;
#18696=PLANE ( 'NONE',  #15782 ) ;
#18734=CARTESIAN_POINT ( 'NONE',  ( 15.45515798858408907, -34.86679772354910511, 6.222782430144768284 ) ) ;
#18809=CARTESIAN_POINT ( 'NONE',  ( -8.789023433377586514, -31.87591480792581322, 13.49878314047843020 ) ) ;
#18855=CARTESIAN_POINT ( 'NONE',  ( -4.228765754682470401, -25.91303510919334485, -15.38236557491807766 ) ) ;
#18869=CARTESIAN_POINT ( 'NONE',  ( -25.00000000000000355, -30.00000000000000000, 1.530808498934191521E-15 ) ) ;
#18880=VERTEX_POINT ( 'NONE', #116 ) ;
#19012=CARTESIAN_POINT ( 'NONE',  ( -18.06522620542768109, -29.74877956674518131, -8.189528952361769143 ) ) ;
#19086=CARTESIAN_POINT ( 'NONE',  ( 28.27451930523357504, -3.452175767011101293, -24.83788945613661880 ) ) ;
#19095=CIRCLE ( 'NONE', #1072, 16.19615242270663558 ) ;
#19123=CARTESIAN_POINT ( 'NONE',  ( -10.70822065730263084, -29.54386645810036782, 10.21044671111158664 ) ) ;
#19133=CARTESIAN_POINT ( 'NONE',  ( 37.25000000000000711, -1.694065894508600678E-18, 1.500000000000000222 ) ) ;
#19141=DIRECTION ( 'NONE',  ( -0.2475719085175093481, -0.000000000000000000, -0.9688695217174488894 ) ) ;
#19143=CARTESIAN_POINT ( 'NONE',  ( -41.00000000000000711, -1.694065894508600678E-18, 0.000000000000000000 ) ) ;
#19173=CARTESIAN_POINT ( 'NONE',  ( -2.112161198359963521, -25.77267402162640408, -15.59357793625674660 ) ) ;
#19214=CARTESIAN_POINT ( 'NONE',  ( -22.00000000000000711, -20.00000000000000000, 2.449293598294706907E-15 ) ) ;
#19222=TOROIDAL_SURFACE ( 'NONE', #9665, 5.000000000000000888, 19.00000000000000000 ) ;
#19285=ORIENTED_EDGE ( 'NONE', *, *, #7792, .F. ) ;
#19336=CARTESIAN_POINT ( 'NONE',  ( -12.53824232977090603, -28.27004406456470775, 13.15159876983787335 ) ) ;
#19346=CARTESIAN_POINT ( 'NONE',  ( -10.77421046970567708, -27.84620353580639218, -14.04190754122875973 ) ) ;
#19370=CIRCLE ( 'NONE', #56541, 19.00000000000000000 ) ;
#19379=CARTESIAN_POINT ( 'NONE',  ( 1.845799476742940870, -28.15607794640831330, -13.84328548073280629 ) ) ;
#19465=CARTESIAN_POINT ( 'NONE',  ( 14.53304282576173634, -29.99999999999999289, 3.713578627762628592 ) ) ;
#19492=EDGE_CURVE ( 'NONE', #31440, #3747, #20821, .T. ) ;
#19493=CYLINDRICAL_SURFACE ( 'NONE', #47249, 1.500000000000000222 ) ;
#19509=CARTESIAN_POINT ( 'NONE',  ( -13.53218314551040002, -34.21215502346704085, -9.055742533982485298 ) ) ;
#19518=CARTESIAN_POINT ( 'NONE',  ( -9.974301738911194093, -29.01869747443885927, -8.904338584474109197 ) ) ;
#19578=ORIENTED_EDGE ( 'NONE', *, *, #51742, .T. ) ;
#19593=CARTESIAN_POINT ( 'NONE',  ( 11.92950489380962331, -32.88714273283137857, -11.67197772324075267 ) ) ;
#19649=DIRECTION ( 'NONE',  ( 1.000000000000000000, -0.000000000000000000, -0.000000000000000000 ) ) ;
#19661=ADVANCED_FACE ( 'NONE', ( #5626 ), #8708, .F. ) ;
#19669=CARTESIAN_POINT ( 'NONE',  ( 4.028938272669588372, -26.74124408001654984, 15.94258242224534960 ) ) ;
#19681=CARTESIAN_POINT ( 'NONE',  ( -12.53824232977091491, -28.27004406456470775, -13.15159876983786980 ) ) ;
#19712=CARTESIAN_POINT ( 'NONE',  ( -1.825668173474439993, -28.16298946971344108, -13.82820292526064776 ) ) ;
#19734=ORIENTED_EDGE ( 'NONE', *, *, #1736, .T. ) ;
#19745=LINE ( 'NONE', #54971, #15878 ) ;
#19754=CARTESIAN_POINT ( 'NONE',  ( -49.96127604611442763, -0.007915161567797545511, -1.618137530678320335 ) ) ;
#19775=EDGE_LOOP ( 'NONE', ( #27765, #17945, #39780, #22475 ) ) ;
#19782=CARTESIAN_POINT ( 'NONE',  ( -16.37486794060187734, -28.33944867960597236, 9.978426449060183501 ) ) ;
#19792=DIRECTION ( 'NONE',  ( 0.000000000000000000, 1.000000000000000000, 0.000000000000000000 ) ) ;
#19793=CARTESIAN_POINT ( 'NONE',  ( 17.33919137821584044, -29.56463768738094089, 9.168593624349419713 ) ) ;
#19800=ORIENTED_EDGE ( 'NONE', *, *, #11614, .F. ) ;
#19829=CARTESIAN_POINT ( 'NONE',  ( -12.31625042011854454, -33.75886355119538962, -10.24605909438320950 ) ) ;
#19834=CARTESIAN_POINT ( 'NONE',  ( 14.05446433506782533, -34.40329588773735736, -8.438602785652603799 ) ) ;
#19845=CARTESIAN_POINT ( 'NONE',  ( -25.00000000000000355, -9.999999999999998224, 1.530808498934191521E-15 ) ) ;
#19855=SURFACE_SIDE_STYLE ('',( #49484 ) ) ;
#19866=DIRECTION ( 'NONE',  ( 0.000000000000000000, -0.000000000000000000, -1.000000000000000000 ) ) ;
#19875=DIRECTION ( 'NONE',  ( 0.000000000000000000, 0.000000000000000000, 1.000000000000000000 ) ) ;
#19888=DIRECTION ( 'NONE',  ( -0.2475719085175098477, 0.000000000000000000, -0.9688695217174486674 ) ) ;
#19911=CARTESIAN_POINT ( 'NONE',  ( -12.96770491601581021, -33.25366259606034447, 10.81293556751078988 ) ) ;
#19950=CARTESIAN_POINT ( 'NONE',  ( -14.48921874744988614, -27.84739049628997876, 11.52341872854555227 ) ) ;
#19954=CARTESIAN_POINT ( 'NONE',  ( -41.00000000000000711, -45.00200000000000244, -4.500000000000000888 ) ) ;
#19975=SURFACE_SIDE_STYLE ('',( #65506 ) ) ;
#19976=CARTESIAN_POINT ( 'NONE',  ( -18.85528480568559573, -29.92804508438502609, 6.903306693652388581 ) ) ;
#19985=CARTESIAN_POINT ( 'NONE',  ( -7.961359079021525176, -27.27258404549933246, -15.08967732372090609 ) ) ;
#20017=CARTESIAN_POINT ( 'NONE',  ( 2.128776824815503677, -26.59425375116049040, -16.16470972310717968 ) ) ;
#20019=CARTESIAN_POINT ( 'NONE',  ( 41.00000000000000711, -25.45369917733758314, 1.516638822270951703 ) ) ;
#20051=CIRCLE ( 'NONE', #11538, 1.500000000000000444 ) ;
#20066=CARTESIAN_POINT ( 'NONE',  ( 49.83768944945995827, -0.03330036048198387055, -3.290779520873021724 ) ) ;
#20081=ORIENTED_EDGE ( 'NONE', *, *, #46210, .F. ) ;
#20095=CARTESIAN_POINT ( 'NONE',  ( -14.06029564544070531, -34.40539544390912141, 8.431086515739542264 ) ) ;
#20104=CIRCLE ( 'NONE', #34984, 3.000000000000000444 ) ;
#20107=CARTESIAN_POINT ( 'NONE',  ( 9.704251177394615624, -29.31945899942111211, 10.96599872320776115 ) ) ;
#20146=TOROIDAL_SURFACE ( 'NONE', #36071, 20.19615242270663558, 4.000000000000000000 ) ;
#20147=CARTESIAN_POINT ( 'NONE',  ( -12.63451720668099476, -33.87771254755882921, -9.962109630950775951 ) ) ;
#20152=CARTESIAN_POINT ( 'NONE',  ( 12.83306155034124707, -29.03814089299731549, -3.459227852999859021 ) ) ;
#20166=EDGE_CURVE ( 'NONE', #48019, #9242, #713, .T. ) ;
#20177=VECTOR ( 'NONE', #49785, 1000.000000000000000 ) ;
#20224=DIRECTION ( 'NONE',  ( 1.000000000000000000, 0.000000000000000000, -0.000000000000000000 ) ) ;
#20279=CARTESIAN_POINT ( 'NONE',  ( 19.22959543997423992, -28.98134239863147599, 5.957279114860654978 ) ) ;
#20281=CARTESIAN_POINT ( 'NONE',  ( 25.00000000000000355, -30.00000000000000000, -4.999999999999999112 ) ) ;
#20282=DIRECTION ( 'NONE',  ( 0.000000000000000000, 0.000000000000000000, 1.000000000000000000 ) ) ;
#20295=CARTESIAN_POINT ( 'NONE',  ( 22.00000000000000711, -20.00000000000000000, 2.449293598294706907E-15 ) ) ;
#20300=CARTESIAN_POINT ( 'NONE',  ( -40.42380607987477958, -25.46069350086627381, -4.500000000000000888 ) ) ;
#20311=CARTESIAN_POINT ( 'NONE',  ( -2.024814117303749494, -26.59886070765378818, -16.15701038285739699 ) ) ;
#20341=CARTESIAN_POINT ( 'NONE',  ( -4.536586326000698222, -28.39263410566653789, -13.35746355085865211 ) ) ;
#20388=DIRECTION ( 'NONE',  ( 0.000000000000000000, 0.000000000000000000, 1.000000000000000000 ) ) ;
#20392=CARTESIAN_POINT ( 'NONE',  ( 49.84017496522046287, -0.03257330535492963808, 2.852477068595666854 ) ) ;
#20394=CARTESIAN_POINT ( 'NONE',  ( -25.00000000000000355, -3.797884998337192286, -24.99999999999999289 ) ) ;
#20428=CARTESIAN_POINT ( 'NONE',  ( -7.016966734453155219, -28.45964332336963665, 10.94381053768247547 ) ) ;
#20440=CARTESIAN_POINT ( 'NONE',  ( 14.27815883903102900, -30.09651741059085595, 4.806648824293995759 ) ) ;
#20442=DIRECTION ( 'NONE',  ( 0.2475719085175094591, 6.192417051524157726E-18, -0.9688695217174487784 ) ) ;
#20476=ORIENTED_EDGE ( 'NONE', *, *, #34591, .F. ) ;
#20483=CARTESIAN_POINT ( 'NONE',  ( -7.228961821833054024, -32.07041743672399292, -13.19626196499568316 ) ) ;
#20488=CARTESIAN_POINT ( 'NONE',  ( 12.19204271345157586, -29.31683997938284136, -5.830637565203153905 ) ) ;
#20561=DIRECTION ( 'NONE',  ( -1.000000000000000000, -0.000000000000000000, -0.000000000000000000 ) ) ;
#20578=CARTESIAN_POINT ( 'NONE',  ( 0.000000000000000000, -29.00000000000000000, 0.000000000000000000 ) ) ;
#20586=EDGE_LOOP ( 'NONE', ( #28194, #60247, #5458, #7411 ) ) ;
#20644=( NAMED_UNIT ( * ) PLANE_ANGLE_UNIT ( ) SI_UNIT ( $, .RADIAN. ) );
#20681=CARTESIAN_POINT ( 'NONE',  ( -12.89187373143240833, -28.36023352766247996, -12.94763553493058339 ) ) ;
#20689=CARTESIAN_POINT ( 'NONE',  ( -14.34460386949389665, -34.50739325218034281, 8.058841881770181459 ) ) ;
#20720=CARTESIAN_POINT ( 'NONE',  ( -41.00000000000000711, 5.493969937218003549E-16, -4.500000000000000888 ) ) ;
#20750=ORIENTED_EDGE ( 'NONE', *, *, #23408, .F. ) ;
#20756=CARTESIAN_POINT ( 'NONE',  ( -5.901743774574147672, -31.73659747722650692, 13.63115424678022158 ) ) ;
#20766=CARTESIAN_POINT ( 'NONE',  ( 11.32820571420733557, -29.68697874620739796, 9.642237626533521677 ) ) ;
#20777=ORIENTED_EDGE ( 'NONE', *, *, #50453, .T. ) ;
#20807=CARTESIAN_POINT ( 'NONE',  ( -0.8753493882257603609, -31.04850208196563344, -14.43082775300592324 ) ) ;
#20812=CARTESIAN_POINT ( 'NONE',  ( 12.69762816655162574, -29.19309327991418357, -4.289906119468183121 ) ) ;
#20820=DIRECTION ( 'NONE',  ( 0.2475719085175098200, -2.922992529533354589E-16, -0.9688695217174487784 ) ) ;
#20821=B_SPLINE_CURVE_WITH_KNOTS ( 'NONE', 3,
 ( #7653, #59186, #32894, #7304, #27589, #63487, #47890, #38218, #28264, #49224, #8305, #2349, #33890, #8629, #24241, #19911, #34846, #9581, #45185, #55155, #34544, #50835, #34218, #13924, #30220, #3978 ),
 .UNSPECIFIED., .F., .F.,
 ( 4, 2, 2, 2, 2, 2, 2, 2, 2, 2, 2, 2, 4 ),
 ( 0.02249411442595698057, 0.02389926644164680827, 0.02530441845733663597, 0.02811472248871628790, 0.02951987450440611213, 0.03092502652009593983, 0.03373533055147559523, 0.03654563458285524369, 0.03795078659854507486, 0.03935593861423490603, 0.04076109062992473026, 0.04216624264561455449, 0.04497654667699420294 ),
 .UNSPECIFIED. ) ;
#20917=CARTESIAN_POINT ( 'NONE',  ( -48.17199526896420991, -0.3660652840184910883, 6.262213226250253228 ) ) ;
#20947=CARTESIAN_POINT ( 'NONE',  ( 0.9972908435452140230, -25.72582856205513835, -15.66294124711422775 ) ) ;
#20948=CARTESIAN_POINT ( 'NONE',  ( 11.20797324838624220, -27.95044230146133657, 13.82289656124155997 ) ) ;
#20965=EDGE_CURVE ( 'NONE', #15192, #46997, #58756, .T. ) ;
#20985=CARTESIAN_POINT ( 'NONE',  ( 11.15801620995752863, -32.62087690405027018, -12.20531625113489227 ) ) ;
#20993=LINE ( 'NONE', #41274, #7504 ) ;
#21028=TOROIDAL_SURFACE ( 'NONE', #41242, 5.000000000000000888, 20.00000000000000000 ) ;
#21030=DIRECTION ( 'NONE',  ( -1.000000000000000000, 0.000000000000000000, -1.224646799147353207E-16 ) ) ;
#21031=CARTESIAN_POINT ( 'NONE',  ( 26.64924965067720564, -3.627973872667549671, 24.95916750106484727 ) ) ;
#21064=CARTESIAN_POINT ( 'NONE',  ( -5.484316184572717745, -28.21670571277722672, 11.61674069750055160 ) ) ;
#21116=CARTESIAN_POINT ( 'NONE',  ( 12.62425547244847124, -33.87255953084252980, 9.995598718700033913 ) ) ;
#21126=CARTESIAN_POINT ( 'NONE',  ( 11.41243050843482187, -29.26822538582705491, -7.243948608349865204 ) ) ;
#21168=FACE_OUTER_BOUND ( 'NONE', #43214, .T. ) ;
#21177=CARTESIAN_POINT ( 'NONE',  ( -25.00000000000000355, -9.999999999999998224, 24.00000000000000000 ) ) ;
#21239=CARTESIAN_POINT ( 'NONE',  ( -16.81745777873098291, -34.49999999816794372, 5.267778333666917945 ) ) ;
#21269=DIRECTION ( 'NONE',  ( 0.000000000000000000, 0.000000000000000000, -1.000000000000000000 ) ) ;
#21279=CARTESIAN_POINT ( 'NONE',  ( 5.446351735594772592, -26.05211744559319342, -15.16580142939698028 ) ) ;
#21302=EDGE_CURVE ( 'NONE', #59550, #3889, #13495, .T. ) ;
#21306=CARTESIAN_POINT ( 'NONE',  ( 43.07244751019904072, -1.315220855092162688, 15.87097690372581837 ) ) ;
#21313=CARTESIAN_POINT ( 'NONE',  ( -16.21117406328131949, -35.00000000000000000, 4.142385751841757724 ) ) ;
#21323=CARTESIAN_POINT ( 'NONE',  ( 9.349182579143132443, -29.24123260035265659, -11.20990699596419127 ) ) ;
#21330=AXIS2_PLACEMENT_3D ( 'NONE', #26917, #47216, #57514 ) ;
#21337=CARTESIAN_POINT ( 'NONE',  ( 25.00000000000000355, -30.00000000000000000, 1.530808498934191521E-15 ) ) ;
#21381=EDGE_CURVE ( 'NONE', #41515, #44894, #54707, .T. ) ;
#21411=CARTESIAN_POINT ( 'NONE',  ( 9.079541994506246994, -32.62122108031978485, 12.39463523794014321 ) ) ;
#21450=AXIS2_PLACEMENT_3D ( 'NONE', #16496, #20820, #10840 ) ;
#21467=CIRCLE ( 'NONE', #53335, 5.000000000000001776 ) ;
#21536=CYLINDRICAL_SURFACE ( 'NONE', #40394, 250.0000000000000000 ) ;
#21561=CARTESIAN_POINT ( 'NONE',  ( -16.21117406328131949, -35.00000000000000000, -4.142385751841763053 ) ) ;
#21625=ORIENTED_EDGE ( 'NONE', *, *, #65363, .T. ) ;
#21658=CARTESIAN_POINT ( 'NONE',  ( 48.36589927958296187, -0.3279091627047653890, -5.494672883103046246 ) ) ;
#21661=EDGE_CURVE ( 'NONE', #14466, #51562, #23811, .T. ) ;
#21676=CARTESIAN_POINT ( 'NONE',  ( 17.91771366450656444, -29.71233038866040133, -8.402389056493886343 ) ) ;
#21683=CARTESIAN_POINT ( 'NONE',  ( -15.66937148611438957, -34.93011823067257637, 5.816432770872767222 ) ) ;
#21702=CARTESIAN_POINT ( 'NONE',  ( -22.00000000000000711, -20.00000000000000000, 1.500000000000002887 ) ) ;
#21755=CARTESIAN_POINT ( 'NONE',  ( 1.749504362522309897, -27.84680466544767796, 12.51149646090675915 ) ) ;
#21881=CARTESIAN_POINT ( 'NONE',  ( -49.83768944945995116, -0.03330036048197439202, 3.290779520873027941 ) ) ;
#21949=CARTESIAN_POINT ( 'NONE',  ( 17.99690872998901270, -28.74566129397117464, -8.126501682513225688 ) ) ;
#21982=EDGE_CURVE ( 'NONE', #25095, #59550, #61782, .T. ) ;
#21983=CARTESIAN_POINT ( 'NONE',  ( 9.704251177394571215, -29.31945899941926115, -10.96599872320825142 ) ) ;
#22056=CARTESIAN_POINT ( 'NONE',  ( 1.730912674848539366E-15, -30.50000000000000000, 14.13397459621556251 ) ) ;
#22057=CARTESIAN_POINT ( 'NONE',  ( 7.742519806647712777, -28.58895386040045494, 10.54525737088725101 ) ) ;
#22145=CARTESIAN_POINT ( 'NONE',  ( -39.58329824467849534, -1.898237318462467682, 19.07749194152998484 ) ) ;
#22193=CARTESIAN_POINT ( 'NONE',  ( -11.91618201078742523, -29.31229682091840871, -6.386286639733476100 ) ) ;
#22226=VERTEX_POINT ( 'NONE', #24503 ) ;
#22228=CARTESIAN_POINT ( 'NONE',  ( -17.34314652423486081, -29.56569286319712475, -9.163921882788894635 ) ) ;
#22242=FACE_OUTER_BOUND ( 'NONE', #44761, .T. ) ;
#22255=ORIENTED_EDGE ( 'NONE', *, *, #40737, .T. ) ;
#22260=CARTESIAN_POINT ( 'NONE',  ( 17.75832895199378214, -29.67262258703657096, 8.626345146652846907 ) ) ;
#22288=CIRCLE ( 'NONE', #52033, 20.19615242270663558 ) ;
#22341=CARTESIAN_POINT ( 'NONE',  ( 18.04777717444645191, -29.74456712077427056, -8.215504029118783080 ) ) ;
#22354=VECTOR ( 'NONE', #2583, 1000.000000000000000 ) ;
#22378=CARTESIAN_POINT ( 'NONE',  ( -0.8584944786142326700, -27.82166925786467004, 12.56635396443958719 ) ) ;
#22401=ORIENTED_EDGE ( 'NONE', *, *, #13158, .T. ) ;
#22438=EDGE_CURVE ( 'NONE', #46997, #15192, #41910, .T. ) ;
#22474=AXIS2_PLACEMENT_3D ( 'NONE', #40065, #19141, #34091 ) ;
#22475=ORIENTED_EDGE ( 'NONE', *, *, #24038, .T. ) ;
#22481=CARTESIAN_POINT ( 'NONE',  ( -25.79281180259794226, -3.718204414137740610, -24.00000000000000355 ) ) ;
#22490=VECTOR ( 'NONE', #7391, 1000.000000000000000 ) ;
#22501=FACE_BOUND ( 'NONE', #46772, .T. ) ;
#22520=ORIENTED_EDGE ( 'NONE', *, *, #20965, .F. ) ;
#22532=CARTESIAN_POINT ( 'NONE',  ( -37.49868115534710711, -2.226531222652248232, 21.71250474234130579 ) ) ;
#22537=ORIENTED_EDGE ( 'NONE', *, *, #55975, .F. ) ;
#22538=CARTESIAN_POINT ( 'NONE',  ( -11.38801898431830040, -29.26006678106167769, -7.242958320505154646 ) ) ;
#22572=CARTESIAN_POINT ( 'NONE',  ( -13.03183108261446144, -30.03462372422786331, -7.545134388565382544 ) ) ;
#22617=DIRECTION ( 'NONE',  ( -0.000000000000000000, -0.000000000000000000, 1.000000000000000000 ) ) ;
#22623=PRODUCT_DEFINITION_CONTEXT ( 'detailed design', #6035, 'design' ) ;
#22639=VECTOR ( 'NONE', #62512, 1000.000000000000000 ) ;
#22698=CARTESIAN_POINT ( 'NONE',  ( 9.372867312212058266, -27.54793913079791068, -14.59713702163757176 ) ) ;
#22713=LINE ( 'NONE', #13050, #37429 ) ;
#22768=ORIENTED_EDGE ( 'NONE', *, *, #32919, .F. ) ;
#22781=CARTESIAN_POINT ( 'NONE',  ( -41.00000000000000711, -25.49198847189178707, 0.7539676769129274314 ) ) ;
#22822=CARTESIAN_POINT ( 'NONE',  ( -48.96282442591977713, -0.2094399512627133919, -1.553366803981108601 ) ) ;
#22867=CARTESIAN_POINT ( 'NONE',  ( -31.45682506574155113, -3.065323467461852136, 24.16565572891780178 ) ) ;
#22906=DIRECTION ( 'NONE',  ( -0.2475719085175093481, -0.000000000000000000, -0.9688695217174488894 ) ) ;
#22943=CARTESIAN_POINT ( 'NONE',  ( 41.00000000000000711, -1.694065894508793271E-18, 4.500000000000001776 ) ) ;
#22965=CARTESIAN_POINT ( 'NONE',  ( -25.00000000000000355, -9.999999999999998224, -24.00000000000000000 ) ) ;
#22984=EDGE_LOOP ( 'NONE', ( #42421, #56525, #43818, #45795, #55295, #53351 ) ) ;
#22990=CARTESIAN_POINT ( 'NONE',  ( 16.10065672031734962, -35.00000000000000000, -4.574893970807972110 ) ) ;
#23110=ORIENTED_EDGE ( 'NONE', *, *, #48806, .T. ) ;
#23131=CARTESIAN_POINT ( 'NONE',  ( -7.278994278378053018, -27.16225867570152275, 15.27062364585564858 ) ) ;
#23135=CARTESIAN_POINT ( 'NONE',  ( -45.36026561873624274, -0.9018867892165756128, 12.73108497882287971 ) ) ;
#23145=VERTEX_POINT ( 'NONE', #42236 ) ;
#23185=CARTESIAN_POINT ( 'NONE',  ( -12.85491158824215141, -29.00000000000000711, -3.284771503683518556 ) ) ;
#23213=VECTOR ( 'NONE', #16631, 1000.000000000000000 ) ;
#23309=CARTESIAN_POINT ( 'NONE',  ( -2.311295102025900494, -30.63172828985306140, -15.19685615870497131 ) ) ;
#23393=ORIENTED_EDGE ( 'NONE', *, *, #1736, .F. ) ;
#23408=EDGE_CURVE ( 'NONE', #41367, #8147, #556, .T. ) ;
#23417=CARTESIAN_POINT ( 'NONE',  ( 33.02316666837520387, -2.861627175174544568, -23.69173491641420171 ) ) ;
#23460=CARTESIAN_POINT ( 'NONE',  ( -8.761386526127953545, -27.42676914488322026, 14.81571904625999103 ) ) ;
#23510=VECTOR ( 'NONE', #13164, 1000.000000000000000 ) ;
#23520=CARTESIAN_POINT ( 'NONE',  ( -3.456075311296388453, -27.96820792850356341, -12.23233986317338129 ) ) ;
#23525=AXIS2_PLACEMENT_3D ( 'NONE', #37118, #61403, #15843 ) ;
#23532=DIRECTION ( 'NONE',  ( 0.000000000000000000, 0.000000000000000000, 1.000000000000000000 ) ) ;
#23612=ORIENTED_EDGE ( 'NONE', *, *, #57402, .F. ) ;
#23722=CARTESIAN_POINT ( 'NONE',  ( 37.25000000000000711, -27.21021009056489603, 4.499999999999997335 ) ) ;
#23804=CARTESIAN_POINT ( 'NONE',  ( -41.00000000000000711, -1.853910857666116187E-16, -1.500000000000000222 ) ) ;
#23810=CARTESIAN_POINT ( 'NONE',  ( -8.639472567037733697, -29.08579227083833629, 11.67554154369881836 ) ) ;
#23811=CIRCLE ( 'NONE', #14238, 3.000000000000000444 ) ;
#23860=CARTESIAN_POINT ( 'NONE',  ( -8.269707202464745777, -26.46746146559253532, -14.47885724100708416 ) ) ;
#23861=ORIENTED_EDGE ( 'NONE', *, *, #58536, .F. ) ;
#23871=CARTESIAN_POINT ( 'NONE',  ( 41.00000000000000711, -1.694065894508600678E-18, 0.000000000000000000 ) ) ;
#23979=CARTESIAN_POINT ( 'NONE',  ( -11.19906371801375577, -32.63487729457269637, -12.17775756912196172 ) ) ;
#23994=EDGE_LOOP ( 'NONE', ( #16254, #28259, #22537, #38419 ) ) ;
#24002=ORIENTED_EDGE ( 'NONE', *, *, #42252, .F. ) ;
#24024=CARTESIAN_POINT ( 'NONE',  ( 41.00000000000000711, -25.03188948156373428, -4.500000000000011546 ) ) ;
#24038=EDGE_CURVE ( 'NONE', #4569, #33520, #25680, .T. ) ;
#24105=ADVANCED_FACE ( 'NONE', ( #1730 ), #6721, .T. ) ;
#24114=ORIENTED_EDGE ( 'NONE', *, *, #52243, .T. ) ;
#24117=CARTESIAN_POINT ( 'NONE',  ( -14.21898193534997290, -33.70038524408893466, 9.575031237889474411 ) ) ;
#24131=DIRECTION ( 'NONE',  ( 0.000000000000000000, 0.000000000000000000, 1.000000000000000000 ) ) ;
#24159=CARTESIAN_POINT ( 'NONE',  ( 6.734959099364806079, -31.93290117444115594, -13.38585010773448580 ) ) ;
#24170=DIRECTION ( 'NONE',  ( -0.000000000000000000, -1.000000000000000000, -0.000000000000000000 ) ) ;
#24175=DIRECTION ( 'NONE',  ( -1.000000000000000000, -0.000000000000000000, -0.000000000000000000 ) ) ;
#24184=SURFACE_STYLE_USAGE ( .BOTH. , #19855 ) ;
#24202=DIRECTION ( 'NONE',  ( -0.2475719085175094869, 0.000000000000000000, -0.9688695217174488894 ) ) ;
#24234=CARTESIAN_POINT ( 'NONE',  ( 17.05023968204110574, -34.50000000000000000, -4.356789313881336057 ) ) ;
#24241=CARTESIAN_POINT ( 'NONE',  ( -11.92921645562187294, -32.88698380610403404, 11.67323352594769936 ) ) ;
#24248=ORIENTED_EDGE ( 'NONE', *, *, #8057, .T. ) ;
#24249=CARTESIAN_POINT ( 'NONE',  ( 0.000000000000000000, -33.00000000000000000, 0.000000000000000000 ) ) ;
#24262=DIRECTION ( 'NONE',  ( 0.000000000000000000, 1.000000000000000000, 0.000000000000000000 ) ) ;
#24276=CIRCLE ( 'NONE', #8333, 1.500000000000000444 ) ;
#24285=CARTESIAN_POINT ( 'NONE',  ( -6.328161288312280419, -31.25458527549038124, -14.40172722985745324 ) ) ;
#24319=CARTESIAN_POINT ( 'NONE',  ( 41.00000000000000711, -1.694065894508600678E-18, 0.000000000000000000 ) ) ;
#24334=ADVANCED_FACE ( 'NONE', ( #65180 ), #60514, .T. ) ;
#24345=CARTESIAN_POINT ( 'NONE',  ( -11.13812830829075473, -32.61426855637730426, -12.21782902109653612 ) ) ;
#24370=CARTESIAN_POINT ( 'NONE',  ( -25.00000000000000355, -30.00000000000000000, -25.00000000000000000 ) ) ;
#24389=CARTESIAN_POINT ( 'NONE',  ( 39.53125591517012083, -1.906753238347150381, -20.35939770057403564 ) ) ;
#24418=CARTESIAN_POINT ( 'NONE',  ( -10.50558643126015923, -29.12101583629321055, 8.365681325885642394 ) ) ;
#24427=DIRECTION ( 'NONE',  ( 0.000000000000000000, 1.000000000000000000, 0.000000000000000000 ) ) ;
#24428=CARTESIAN_POINT ( 'NONE',  ( -16.02805653289875920, -29.20913999211457224, 10.57890313540342220 ) ) ;
#24477=CARTESIAN_POINT ( 'NONE',  ( -14.34460386949599631, -34.50739325218108888, -8.058841881767305537 ) ) ;
#24482=CARTESIAN_POINT ( 'NONE',  ( 1.749504362522309897, -27.84680466544767796, -12.51149646090675915 ) ) ;
#24503=CARTESIAN_POINT ( 'NONE',  ( -25.00000000000000355, -9.999999999999998224, 25.00000000000000000 ) ) ;
#24570=EDGE_CURVE ( 'NONE', #16604, #31040, #38859, .T. ) ;
#24573=DIRECTION ( 'NONE',  ( 0.000000000000000000, 1.000000000000000000, 0.000000000000000000 ) ) ;
#24618=CARTESIAN_POINT ( 'NONE',  ( -7.613843340947280325, -31.56230424472762053, -13.96789312046469789 ) ) ;
#24640=ORIENTED_EDGE ( 'NONE', *, *, #28667, .F. ) ;
#24643=CARTESIAN_POINT ( 'NONE',  ( -2.534465382079141182, -26.62629929685679997, 16.11622222973024421 ) ) ;
#24651=ADVANCED_FACE ( 'NONE', ( #2970 ), #21028, .T. ) ;
#24656=AXIS2_PLACEMENT_3D ( 'NONE', #28946, #49255, #39235 ) ;
#24674=B_SPLINE_CURVE_WITH_KNOTS ( 'NONE', 3,
 ( #5692, #25962, #56196, #30592, #20300, #46247 ),
 .UNSPECIFIED., .F., .F.,
 ( 4, 2, 4 ),
 ( 0.006113759649309998857, 0.008271820019583001060, 0.01042988038985600413 ),
 .UNSPECIFIED. ) ;
#24686=CARTESIAN_POINT ( 'NONE',  ( -11.87635721007226053, -32.86858074101943572, -11.71246211286171857 ) ) ;
#24715=B_SPLINE_CURVE_WITH_KNOTS ( 'NONE', 3,
 ( #14611, #39579, #9301, #3718, #38604, #64508, #43923, #38935, #48925, #49893, #28954, #59222, #23979, #28299, #4345, #24618, #44239, #24285, #34893, #18339, #59540, #23309, #13971, #34261, #8998, #65178 ),
 .UNSPECIFIED., .F., .F.,
 ( 4, 2, 2, 2, 2, 2, 2, 2, 2, 2, 2, 2, 4 ),
 ( 0.000000000000000000, 0.002759437753103677511, 0.004139156629655517568, 0.005518875506207357624, 0.006898594382759197681, 0.008278313259311036870, 0.01103775101241471525, 0.01379718876551839189, 0.01517690764207022848, 0.01655662651862206680, 0.01931606427172574345, 0.02069578314827758003, 0.02207550202482942009 ),
 .UNSPECIFIED. ) ;
#24739=CARTESIAN_POINT ( 'NONE',  ( 14.80527133490690694, -33.90607016887848602, 8.874040421128851719 ) ) ;
#24763=CARTESIAN_POINT ( 'NONE',  ( -15.04954985558960878, -34.74586518154888637, 6.983850705393018998 ) ) ;
#24776=CARTESIAN_POINT ( 'NONE',  ( 13.56792483471932798, -30.10715271124615455, 6.611461891173466832 ) ) ;
#24819=ADVANCED_FACE ( 'NONE', ( #9228, #50148 ), #43341, .F. ) ;
#24826=CARTESIAN_POINT ( 'NONE',  ( 9.075728589825974524, -28.84360970496360466, -9.643933591119377979 ) ) ;
#24857=DIRECTION ( 'NONE',  ( 0.000000000000000000, 0.000000000000000000, 1.000000000000000000 ) ) ;
#24936=ORIENTED_EDGE ( 'NONE', *, *, #32639, .T. ) ;
#24955=CARTESIAN_POINT ( 'NONE',  ( 12.41715713833625045, -27.32744910944862227, 12.80873342738428278 ) ) ;
#24956=PLANE ( 'NONE',  #54249 ) ;
#24966=AXIS2_PLACEMENT_3D ( 'NONE', #10040, #15352, #14667 ) ;
#24973=DIRECTION ( 'NONE',  ( 0.000000000000000000, -0.000000000000000000, 1.000000000000000000 ) ) ;
#24977=FILL_AREA_STYLE_COLOUR ( '', #46743 ) ;
#24994=ADVANCED_FACE ( 'NONE', ( #22501, #54071, #27813 ), #28792, .F. ) ;
#25017=CARTESIAN_POINT ( 'NONE',  ( -0.5153900578009920075, -26.55329395651783031, -16.22445808467987050 ) ) ;
#25062=CARTESIAN_POINT ( 'NONE',  ( 49.66779747649341914, -0.06758380666731210462, 4.082965791224114405 ) ) ;
#25067=CARTESIAN_POINT ( 'NONE',  ( 16.25676674326443560, -34.36623312464853797, 6.550321452246427256 ) ) ;
#25089=DIRECTION ( 'NONE',  ( 0.000000000000000000, 0.000000000000000000, -1.000000000000000000 ) ) ;
#25092=CARTESIAN_POINT ( 'NONE',  ( -17.92531974009704498, -28.72851451116432031, 8.222150688345376324 ) ) ;
#25095=VERTEX_POINT ( 'NONE', #27043 ) ;
#25102=CARTESIAN_POINT ( 'NONE',  ( 8.295782569430503628, -27.33295754267858158, 14.98640435465113541 ) ) ;
#25129=DIRECTION ( 'NONE',  ( 0.000000000000000000, 0.000000000000000000, 1.000000000000000000 ) ) ;
#25138=CARTESIAN_POINT ( 'NONE',  ( 10.63582125257018163, -33.14335888457333112, 11.52436878476033932 ) ) ;
#25141=CARTESIAN_POINT ( 'NONE',  ( -1.754394376714002002, -31.09667363889299097, -14.37851519254829391 ) ) ;
#25146=CARTESIAN_POINT ( 'NONE',  ( 12.57831868240780082, -29.25370879966640203, -4.768001503383415773 ) ) ;
#25231=EDGE_CURVE ( 'NONE', #34941, #37781, #20051, .T. ) ;
#25256=ORIENTED_EDGE ( 'NONE', *, *, #46210, .T. ) ;
#25262=CARTESIAN_POINT ( 'NONE',  ( 19.41740522748897391, -28.99999999999999289, 5.485033347092790557 ) ) ;
#25301=EDGE_CURVE ( 'NONE', #53510, #32724, #17727, .T. ) ;
#25318=ORIENTED_EDGE ( 'NONE', *, *, #14981, .T. ) ;
#25324=ORIENTED_EDGE ( 'NONE', *, *, #65588, .T. ) ;
#25329=CARTESIAN_POINT ( 'NONE',  ( 6.272189122743162315, -31.23296902231907879, -14.43357722546949162 ) ) ;
#25332=DIRECTION ( 'NONE',  ( 0.000000000000000000, 0.000000000000000000, 1.000000000000000000 ) ) ;
#25352=DIRECTION ( 'NONE',  ( 1.000000000000000000, 0.000000000000000000, -0.000000000000000000 ) ) ;
#25357=DIRECTION ( 'NONE',  ( -1.000000000000000000, 0.000000000000000000, -0.000000000000000000 ) ) ;
#25377=CARTESIAN_POINT ( 'NONE',  ( -33.05588761701186939, -2.860689001541065313, -23.72276540370178566 ) ) ;
#25407=CARTESIAN_POINT ( 'NONE',  ( -41.00000000000000711, -45.00200000000000244, 4.499999999999997335 ) ) ;
#25408=CARTESIAN_POINT ( 'NONE',  ( -8.110750208426855679, -28.65453171997180348, 10.34333599818648608 ) ) ;
#25420=CARTESIAN_POINT ( 'NONE',  ( 5.786001662380197530, -26.94056086434354924, 15.63186719136363401 ) ) ;
#25428=ORIENTED_EDGE ( 'NONE', *, *, #55975, .T. ) ;
#25467=CARTESIAN_POINT ( 'NONE',  ( 12.80904563207495350, -29.07871018746070391, -3.648338481107154863 ) ) ;
#25480=CARTESIAN_POINT ( 'NONE',  ( 16.21117406328131949, -35.00000000000000000, 4.142385751841762165 ) ) ;
#25493=AXIS2_PLACEMENT_3D ( 'NONE', #16580, #10927, #31214 ) ;
#25587=ORIENTED_EDGE ( 'NONE', *, *, #21381, .F. ) ;
#25597=CARTESIAN_POINT ( 'NONE',  ( 17.69916095700584435, -28.67478364583445938, 8.521665482016091531 ) ) ;
#25621=CARTESIAN_POINT ( 'NONE',  ( -5.041025311761524463, -26.84022127302798921, 15.79220748139831265 ) ) ;
#25627=CARTESIAN_POINT ( 'NONE',  ( 0.000000000000000000, 244.9489742783177917, -23.99999999999999289 ) ) ;
#25644=DIRECTION ( 'NONE',  ( 1.000000000000000000, -0.000000000000000000, -0.000000000000000000 ) ) ;
#25663=CARTESIAN_POINT ( 'NONE',  ( -10.70822065730027184, -29.54386645810234313, -10.21044671110655777 ) ) ;
#25680=LINE ( 'NONE', #426, #2786 ) ;
#25712=CARTESIAN_POINT ( 'NONE',  ( 48.39008813825011401, -0.3233266992476154233, -8.863930066451532142 ) ) ;
#25717=CARTESIAN_POINT ( 'NONE',  ( 7.188828048480045751, -31.44854185097605637, 14.13838964164171585 ) ) ;
#25748=CARTESIAN_POINT ( 'NONE',  ( -8.269707202464745777, -26.46746146559253532, 14.47885724100708416 ) ) ;
#25759=CARTESIAN_POINT ( 'NONE',  ( 17.02556425888772296, -29.48112685930881227, 9.540979227922154138 ) ) ;
#25799=CARTESIAN_POINT ( 'NONE',  ( 15.04427341497070714, -34.74416750921062658, 6.992747701482930012 ) ) ;
#25802=CARTESIAN_POINT ( 'NONE',  ( -13.24204686117535879, -34.10419274375227872, -9.367294588217838225 ) ) ;
#25807=CARTESIAN_POINT ( 'NONE',  ( 15.04222346523121168, -34.74354600359600909, -6.996510958921167145 ) ) ;
#25880=FACE_OUTER_BOUND ( 'NONE', #45381, .T. ) ;
#25927=CARTESIAN_POINT ( 'NONE',  ( -45.77739315166650869, -0.8244463642989293684, -12.03838484699752875 ) ) ;
#25930=VERTEX_POINT ( 'NONE', #16802 ) ;
#25939=EDGE_CURVE ( 'NONE', #38363, #16604, #55818, .T. ) ;
#25957=ADVANCED_FACE ( 'NONE', ( #32087, #48641 ), #43972, .F. ) ;
#25962=CARTESIAN_POINT ( 'NONE',  ( -37.91369172636191820, -26.91879662985438415, -4.500000000000000888 ) ) ;
#25963=CARTESIAN_POINT ( 'NONE',  ( 3.967932057708486671, -25.89885127696171452, -15.40358068932206237 ) ) ;
#25976=CLOSED_SHELL ( 'NONE', ( #44643, #48558, #19661, #49991, #41586, #24334, #121, #36034, #56988, #30685, #43062, #24819, #53057, #24105, #59164, #3853, #49242, #5907, #28079, #16221, #60409, #50074, #52039, #24651, #43527, #52939, #48320, #35051, #10833, #4790, #40205, #57600, #34532, #50567, #14351, #16199, #15692, #33869, #48533, #32955, #51344, #35186, #43275, #25957, #24994, #63281, #64931, #11328, #57523, #8437, #49612, #14855, #12672, #44814, #63865, #1709, #51455, #30245 ) ) ;
#25986=CARTESIAN_POINT ( 'NONE',  ( 47.72075422404364531, -0.4543357781461463962, -7.770873616088282532 ) ) ;
#25998=CARTESIAN_POINT ( 'NONE',  ( 37.25000000000000000, -27.41745588273159839, 3.011965929904362405 ) ) ;
#26002=CARTESIAN_POINT ( 'NONE',  ( 10.20102756488483209, -27.72270395345653782, -14.27139701651662129 ) ) ;
#26047=CARTESIAN_POINT ( 'NONE',  ( 49.02672294760360927, -0.1966872720628251858, -6.919866740913554359 ) ) ;
#26081=CARTESIAN_POINT ( 'NONE',  ( 6.734959099364806079, -31.93290117444115594, 13.38585010773448580 ) ) ;
#26091=CARTESIAN_POINT ( 'NONE',  ( 18.18435566811206527, -29.77699652454509760, 8.006764386360600838 ) ) ;
#26135=CARTESIAN_POINT ( 'NONE',  ( 7.742519806647712777, -28.58895386040138220, -10.54525737088771287 ) ) ;
#26167=ORIENTED_EDGE ( 'NONE', *, *, #37311, .F. ) ;
#26246=CARTESIAN_POINT ( 'NONE',  ( -12.92674250727295870, -33.23908083897963905, -10.84893670414234279 ) ) ;
#26257=CARTESIAN_POINT ( 'NONE',  ( -13.26546321032140163, -27.53582555932709397, 12.33704161722047488 ) ) ;
#26299=ORIENTED_EDGE ( 'NONE', *, *, #6034, .F. ) ;
#26301=CARTESIAN_POINT ( 'NONE',  ( 48.96282442591977713, -0.2094399512627206916, 1.553366803981121480 ) ) ;
#26316=CARTESIAN_POINT ( 'NONE',  ( 14.79723931605636444, -33.90329588773487757, -8.884483617263549959 ) ) ;
#26373=ORIENTED_EDGE ( 'NONE', *, *, #9872, .T. ) ;
#26391=CARTESIAN_POINT ( 'NONE',  ( 5.911253750797971662, -28.27393032148221863, 11.47047724608643371 ) ) ;
#26420=DIRECTION ( 'NONE',  ( 0.000000000000000000, 0.000000000000000000, 1.000000000000000000 ) ) ;
#26423=CARTESIAN_POINT ( 'NONE',  ( -25.00000000000000355, -28.99999999999999645, 1.530808498934191521E-15 ) ) ;
#26435=CARTESIAN_POINT ( 'NONE',  ( -25.00000000000000355, -9.999999999999998224, 24.00000000000000000 ) ) ;
#26448=DIRECTION ( 'NONE',  ( -0.000000000000000000, 0.000000000000000000, 1.000000000000000000 ) ) ;
#26470=ORIENTED_EDGE ( 'NONE', *, *, #21661, .T. ) ;
#26509=ORIENTED_EDGE ( 'NONE', *, *, #57969, .T. ) ;
#26598=CARTESIAN_POINT ( 'NONE',  ( -14.48921874744988614, -27.84739049628998231, -11.52341872854555405 ) ) ;
#26599=CARTESIAN_POINT ( 'NONE',  ( 16.79789036561813020, -29.41979974037718648, 9.796743230926852064 ) ) ;
#26603=VERTEX_POINT ( 'NONE', #50120 ) ;
#26604=DIRECTION ( 'NONE',  ( -1.000000000000000000, -0.000000000000000000, -0.000000000000000000 ) ) ;
#26619=CIRCLE ( 'NONE', #48955, 3.999999999999999556 ) ;
#26624=CARTESIAN_POINT ( 'NONE',  ( 45.77110135055801265, -0.8256172497425009471, -12.04909734191306114 ) ) ;
#26641=CARTESIAN_POINT ( 'NONE',  ( 16.93571557946454931, -34.49999999976442666, -4.804977935186947491 ) ) ;
#26682=EDGE_CURVE ( 'NONE', #22226, #64219, #49154, .T. ) ;
#26726=CARTESIAN_POINT ( 'NONE',  ( -2.112161198359963521, -25.77267402162640408, 15.59357793625674660 ) ) ;
#26736=FACE_OUTER_BOUND ( 'NONE', #20586, .T. ) ;
#26782=CIRCLE ( 'NONE', #63954, 20.19615242270663558 ) ;
#26795=DIRECTION ( 'NONE',  ( 1.000000000000000000, -0.000000000000000000, -0.000000000000000000 ) ) ;
#26801=DIRECTION ( 'NONE',  ( -1.000000000000000000, -0.000000000000000000, -0.000000000000000000 ) ) ;
#26852=EDGE_LOOP ( 'NONE', ( #5607, #3040, #31290, #15422 ) ) ;
#26857=CARTESIAN_POINT ( 'NONE',  ( -49.02672294760359506, -0.1966872720628178584, 6.919866740913558800 ) ) ;
#26896=EDGE_CURVE ( 'NONE', #58655, #37233, #39297, .T. ) ;
#26917=CARTESIAN_POINT ( 'NONE',  ( -25.00000000000000355, -9.999999999999998224, -5.000000000000000888 ) ) ;
#26936=CARTESIAN_POINT ( 'NONE',  ( 15.64771680208055749, -28.15000396670248151, -10.66347899870799942 ) ) ;
#26956=ORIENTED_EDGE ( 'NONE', *, *, #34591, .T. ) ;
#26960=CYLINDRICAL_SURFACE ( 'NONE', #5665, 1.500000000000000444 ) ;
#26969=VERTEX_POINT ( 'NONE', #45045 ) ;
#26976=CARTESIAN_POINT ( 'NONE',  ( 37.25000000000000711, -27.21021009056489603, 4.499999999999997335 ) ) ;
#26982=CARTESIAN_POINT ( 'NONE',  ( 11.58535936493772311, -28.03978107659439090, -13.63905399333256341 ) ) ;
#27003=VECTOR ( 'NONE', #26795, 1000.000000000000000 ) ;
#27043=CARTESIAN_POINT ( 'NONE',  ( -41.00000000000000711, -25.03188948156373073, -4.500000000000008882 ) ) ;
#27057=CARTESIAN_POINT ( 'NONE',  ( -1.704253825401055966, -31.09323697348121129, 14.38225808330797584 ) ) ;
#27125=VERTEX_POINT ( 'NONE', #15744 ) ;
#27143=CARTESIAN_POINT ( 'NONE',  ( -43.04762206662383761, -1.319502909267362467, 15.89732852394791784 ) ) ;
#27150=ORIENTED_EDGE ( 'NONE', *, *, #27450, .T. ) ;
#27184=CARTESIAN_POINT ( 'NONE',  ( -49.13724917365555456, -0.1745483773780783232, 6.524050439336994245 ) ) ;
#27219=CARTESIAN_POINT ( 'NONE',  ( 41.00000000000000711, -25.30020925422648048, 3.022492086418942847 ) ) ;
#27223=CARTESIAN_POINT ( 'NONE',  ( -37.25000000000000711, -20.00000000000000000, 2.449293598294706907E-15 ) ) ;
#27237=CONICAL_SURFACE ( 'NONE', #38916, 15.00000000000000000, 0.5235987755983000369 ) ;
#27267=ORIENTED_EDGE ( 'NONE', *, *, #60811, .F. ) ;
#27271=APPLICATION_CONTEXT ( 'automotive_design' ) ;
#27291=CARTESIAN_POINT ( 'NONE',  ( 11.89229108778294908, -32.87417574757987637, -11.69979538107606487 ) ) ;
#27367=CARTESIAN_POINT ( 'NONE',  ( 10.57252189908326301, -33.12087690403964046, 11.56547414815872088 ) ) ;
#27450=EDGE_CURVE ( 'NONE', #54224, #27125, #50045, .T. ) ;
#27456=CARTESIAN_POINT ( 'NONE',  ( -25.00000000000000355, -30.00000000000000000, 25.00000000000000000 ) ) ;
#27463=EDGE_CURVE ( 'NONE', #16604, #31565, #11307, .T. ) ;
#27484=ORIENTED_EDGE ( 'NONE', *, *, #8280, .T. ) ;
#27501=CARTESIAN_POINT ( 'NONE',  ( -25.00000000000000355, -3.797884998337192286, 24.99999999999999289 ) ) ;
#27540=DIRECTION ( 'NONE',  ( -0.2475719085175094869, 0.000000000000000000, -0.9688695217174488894 ) ) ;
#27556=CARTESIAN_POINT ( 'NONE',  ( 16.66082797316812503, -33.00000000000000000, -4.257284274447485473 ) ) ;
#27574=CARTESIAN_POINT ( 'NONE',  ( -25.00000000000000355, -30.00000000000000000, -25.00000000000000000 ) ) ;
#27589=CARTESIAN_POINT ( 'NONE',  ( -2.311295102010213931, -30.63172828985172202, 15.19685615870658602 ) ) ;
#27625=CARTESIAN_POINT ( 'NONE',  ( 15.96337567072090380, -34.98223374851986023, -4.998641903493608041 ) ) ;
#27695=CARTESIAN_POINT ( 'NONE',  ( 14.81496943876074290, -34.66917994667981162, 7.369609160621835464 ) ) ;
#27699=FACE_OUTER_BOUND ( 'NONE', #11, .T. ) ;
#27718=ORIENTED_EDGE ( 'NONE', *, *, #31291, .F. ) ;
#27738=CARTESIAN_POINT ( 'NONE',  ( -41.00000000000000711, -1.853910857666116187E-16, -1.500000000000000222 ) ) ;
#27749=CARTESIAN_POINT ( 'NONE',  ( 1.744217550874541445, -31.08480052993808229, 14.39239673296416377 ) ) ;
#27759=CARTESIAN_POINT ( 'NONE',  ( 37.25000000000000711, -27.21021009056489248, -4.500000000000000888 ) ) ;
#27765=ORIENTED_EDGE ( 'NONE', *, *, #17577, .F. ) ;
#27793=CARTESIAN_POINT ( 'NONE',  ( -46.52334308975180477, -0.6843348755673336337, -10.64746346056990767 ) ) ;
#27794=EDGE_CURVE ( 'NONE', #37233, #58655, #2252, .T. ) ;
#27813=FACE_BOUND ( 'NONE', #65535, .T. ) ;
#27841=CARTESIAN_POINT ( 'NONE',  ( -49.43099673984272613, -0.1154732602011075832, 5.319553669056252154 ) ) ;
#27848=CARTESIAN_POINT ( 'NONE',  ( -17.03240540343445630, -28.50880493221823286, -9.306303259374256953 ) ) ;
#27854=AXIS2_PLACEMENT_3D ( 'NONE', #65235, #7841, #28118 ) ;
#27897=CARTESIAN_POINT ( 'NONE',  ( -37.25000000000000711, -45.00200000000000244, 4.499999999999997335 ) ) ;
#27921=CARTESIAN_POINT ( 'NONE',  ( -18.83018139755648335, -28.92741097219609969, -6.858339499770067960 ) ) ;
#27954=FACE_OUTER_BOUND ( 'NONE', #57995, .T. ) ;
#27964=CARTESIAN_POINT ( 'NONE',  ( -41.00000000000000711, -45.00200000000000244, -4.500000000000000888 ) ) ;
#27975=CARTESIAN_POINT ( 'NONE',  ( 6.013273758134695335, -31.75304111242975580, -13.61309608153482031 ) ) ;
#28012=CARTESIAN_POINT ( 'NONE',  ( 4.028938272669574161, -26.74124408001654629, -15.94258242224534960 ) ) ;
#28045=CARTESIAN_POINT ( 'NONE',  ( 15.96609733983705226, -34.98269025770574103, 4.990963945245213473 ) ) ;
#28068=ORIENTED_EDGE ( 'NONE', *, *, #1547, .T. ) ;
#28079=ADVANCED_FACE ( 'NONE', ( #43079 ), #58743, .T. ) ;
#28100=EDGE_CURVE ( 'NONE', #50924, #38752, #32441, .T. ) ;
#28118=DIRECTION ( 'NONE',  ( 0.000000000000000000, 0.000000000000000000, 1.000000000000000000 ) ) ;
#28128=CARTESIAN_POINT ( 'NONE',  ( -4.228765754682471290, -26.75056327283501290, 15.92880586833495649 ) ) ;
#28134=CARTESIAN_POINT ( 'NONE',  ( -48.99862351417108641, -0.2022747408561963445, 1.593306619454956108 ) ) ;
#28175=CARTESIAN_POINT ( 'NONE',  ( -44.86048679285934782, -0.9948977233718158120, -15.27141897285095240 ) ) ;
#28193=DIRECTION ( 'NONE',  ( 0.000000000000000000, 0.000000000000000000, 1.000000000000000000 ) ) ;
#28194=ORIENTED_EDGE ( 'NONE', *, *, #31723, .F. ) ;
#28207=CARTESIAN_POINT ( 'NONE',  ( -41.00000000000000000, -25.34319448863032065, -3.012683490291699240 ) ) ;
#28252=CARTESIAN_POINT ( 'NONE',  ( -41.00000000000000711, -1.694065894508600678E-18, 1.500000000000000222 ) ) ;
#28254=DIRECTION ( 'NONE',  ( 0.000000000000000000, 0.000000000000000000, 1.000000000000000000 ) ) ;
#28259=ORIENTED_EDGE ( 'NONE', *, *, #42252, .T. ) ;
#28263=CARTESIAN_POINT ( 'NONE',  ( 25.00000000000000355, -3.797884998337192286, 24.99999999999999289 ) ) ;
#28264=CARTESIAN_POINT ( 'NONE',  ( -6.328161288300638176, -31.25458527548780907, 14.40172722986095977 ) ) ;
#28289=ORIENTED_EDGE ( 'NONE', *, *, #20166, .T. ) ;
#28298=CARTESIAN_POINT ( 'NONE',  ( 12.62425547244439095, -33.87255953084102345, -9.995598718703821106 ) ) ;
#28299=CARTESIAN_POINT ( 'NONE',  ( -9.668839327565212471, -32.14098936784623106, -13.07247934321342342 ) ) ;
#28343=CARTESIAN_POINT ( 'NONE',  ( -37.25000000000000711, -1.694065894508793271E-18, 4.500000000000001776 ) ) ;
#28347=ORIENTED_EDGE ( 'NONE', *, *, #53667, .F. ) ;
#28361=CARTESIAN_POINT ( 'NONE',  ( 14.32183389819027930, -34.49933334076765590, 8.089813643623637418 ) ) ;
#28382=EDGE_CURVE ( 'NONE', #34331, #40350, #34114, .T. ) ;
#28438=CARTESIAN_POINT ( 'NONE',  ( 1.074417311476293380, -26.55384113566742599, 16.22365110280896161 ) ) ;
#28452=AXIS2_PLACEMENT_3D ( 'NONE', #32046, #57676, #1813 ) ;
#28454=LINE ( 'NONE', #18167, #50796 ) ;
#28480=CARTESIAN_POINT ( 'NONE',  ( -31.50196089333760696, -3.063567359192253647, -24.19471064305901464 ) ) ;
#28490=CARTESIAN_POINT ( 'NONE',  ( -0.5153900578009965594, -25.72562925869133821, -15.66323518044676000 ) ) ;
#28540=DIRECTION ( 'NONE',  ( 0.000000000000000000, 1.000000000000000000, 0.000000000000000000 ) ) ;
#28590=ORIENTED_EDGE ( 'NONE', *, *, #1547, .F. ) ;
#28592=ORIENTED_EDGE ( 'NONE', *, *, #60811, .T. ) ;
#28609=EDGE_LOOP ( 'NONE', ( #59875, #48645, #23393, #51218 ) ) ;
#28667=EDGE_CURVE ( 'NONE', #38752, #9242, #40535, .T. ) ;
#28682=CARTESIAN_POINT ( 'NONE',  ( 12.85491158824215496, -28.99999999999999645, 3.284771503683511007 ) ) ;
#28718=DIRECTION ( 'NONE',  ( 1.000000000000000000, -0.000000000000000000, -0.000000000000000000 ) ) ;
#28731=EDGE_LOOP ( 'NONE', ( #17563, #64609, #28945, #43216 ) ) ;
#28759=CARTESIAN_POINT ( 'NONE',  ( 25.00000000000000355, -30.00000000000000000, 1.530808498934191521E-15 ) ) ;
#28769=CARTESIAN_POINT ( 'NONE',  ( -12.89187373143239945, -28.36023352766247996, 12.94763553493058872 ) ) ;
#28792=PLANE ( 'NONE',  #38062 ) ;
#28802=CIRCLE ( 'NONE', #17125, 250.0000000000000000 ) ;
#28826=CARTESIAN_POINT ( 'NONE',  ( -8.775649586809111113, -28.78513225414021903, -9.890132258253695241 ) ) ;
#28877=CARTESIAN_POINT ( 'NONE',  ( 41.00000000000000711, -25.03188948156373783, 4.499999999999997335 ) ) ;
#28945=ORIENTED_EDGE ( 'NONE', *, *, #37212, .T. ) ;
#28946=CARTESIAN_POINT ( 'NONE',  ( 37.25000000000000711, -20.00000000000000000, 2.449293598294706907E-15 ) ) ;
#28954=CARTESIAN_POINT ( 'NONE',  ( -12.96770491602036834, -33.25366259606196451, -10.81293556750676466 ) ) ;
#29047=ORIENTED_EDGE ( 'NONE', *, *, #44495, .T. ) ;
#29073=VECTOR ( 'NONE', #29837, 1000.000000000000000 ) ;
#29115=CARTESIAN_POINT ( 'NONE',  ( -1.806230668642147652, -30.59323697348071747, 15.24264478004184120 ) ) ;
#29167=CARTESIAN_POINT ( 'NONE',  ( 7.310206959902322055, -26.30114832292194649, -14.76431686918209785 ) ) ;
#29194=LINE ( 'NONE', #38506, #54988 ) ;
#29236=CARTESIAN_POINT ( 'NONE',  ( 16.45009115226350005, -34.41505313721356885, -6.130398315945338794 ) ) ;
#29304=CARTESIAN_POINT ( 'NONE',  ( 5.029029651858286876, -26.84634345473923034, 15.78007771861068775 ) ) ;
#29310=CARTESIAN_POINT ( 'NONE',  ( -6.997870572558777091, -27.10943569200529524, -15.36011607788393540 ) ) ;
#29320=AXIS2_PLACEMENT_3D ( 'NONE', #62917, #42966, #41653 ) ;
#29328=VERTEX_POINT ( 'NONE', #23804 ) ;
#29340=CARTESIAN_POINT ( 'NONE',  ( -7.103478058731402811, -31.43429545818153414, -14.15162322622638946 ) ) ;
#29368=TOROIDAL_SURFACE ( 'NONE', #9318, 20.19615242270663558, 4.000000000000000000 ) ;
#29375=EDGE_CURVE ( 'NONE', #29328, #61621, #33795, .T. ) ;
#29382=CARTESIAN_POINT ( 'NONE',  ( 37.49868115534709290, -2.226531222652221143, -21.71250474234130579 ) ) ;
#29420=ORIENTED_EDGE ( 'NONE', *, *, #11614, .T. ) ;
#29423=CARTESIAN_POINT ( 'NONE',  ( -8.269707202464745777, -27.33416996378174701, 14.97774446421776240 ) ) ;
#29464=CARTESIAN_POINT ( 'NONE',  ( -7.119438362040798829, -32.04078451673858297, -13.23628618373588317 ) ) ;
#29494=EDGE_LOOP ( 'NONE', ( #58214, #6878, #16170, #61538 ) ) ;
#29526=AXIS2_PLACEMENT_3D ( 'NONE', #48239, #58527, #28254 ) ;
#29537=CARTESIAN_POINT ( 'NONE',  ( 15.08189101924309128, -34.00125857029148335, -8.507794521698972545 ) ) ;
#29628=CARTESIAN_POINT ( 'NONE',  ( 37.25000000000000711, -20.00000000000000000, -1.499999999999998002 ) ) ;
#29650=CARTESIAN_POINT ( 'NONE',  ( -9.369086346427730305, -29.24458096581343725, -11.21746676167145473 ) ) ;
#29683=SHAPE_REPRESENTATION ( 'Inner cradle housing', ( #24966 ), #5855 ) ;
#29697=CARTESIAN_POINT ( 'NONE',  ( -49.84017496522046997, -0.03257330535494378648, -2.852477068595663301 ) ) ;
#29701=CARTESIAN_POINT ( 'NONE',  ( 17.05023968204110929, -34.50000000000000000, 4.356789313881321846 ) ) ;
#29726=CARTESIAN_POINT ( 'NONE',  ( -17.34314652423584491, -28.58740822003687754, 8.955725788651514918 ) ) ;
#29736=CARTESIAN_POINT ( 'NONE',  ( 0.000000000000000000, -29.00000000000000000, 0.000000000000000000 ) ) ;
#29737=CARTESIAN_POINT ( 'NONE',  ( 4.958255736529285862, -30.98164499407798189, 14.76282592124280058 ) ) ;
#29777=MECHANICAL_DESIGN_GEOMETRIC_PRESENTATION_REPRESENTATION('',(#18093),#14920);
#29779=CARTESIAN_POINT ( 'NONE',  ( -10.63305928498245301, -33.14245637257819510, -11.52579945307858011 ) ) ;
#29785=CARTESIAN_POINT ( 'NONE',  ( -5.484316184572717745, -28.21670571277537221, -11.61674069750055160 ) ) ;
#29837=DIRECTION ( 'NONE',  ( 1.000000000000000000, -0.000000000000000000, -0.000000000000000000 ) ) ;
#29891=( BOUNDED_SURFACE ( )  B_SPLINE_SURFACE ( 3, 2, ( 
 ( #31833, #23185, #57135 ),
 ( #11561, #1923, #37152 ),
 ( #47483, #12529, #37493 ),
 ( #52148, #6597, #57462 ),
 ( #11885, #38135, #32162 ),
 ( #12219, #53118, #52486 ),
 ( #32809, #32486, #27848 ),
 ( #6920, #22193, #42451 ),
 ( #2611, #52792, #7221 ),
 ( #2259, #22538, #42802 ),
 ( #63092, #43125, #63403 ),
 ( #58444, #12875, #33154 ),
 ( #8220, #19518, #34125 ),
 ( #54099, #28826, #3902 ),
 ( #9186, #39783, #59745 ),
 ( #29464, #54768, #38809 ),
 ( #64075, #65041, #23860 ),
 ( #39119, #63727, #49463 ),
 ( #55071, #29785, #8537 ),
 ( #59108, #49766, #64704 ),
 ( #58793, #23520, #18855 ),
 ( #18207, #49135, #13211 ),
 ( #13517, #43448, #19173 ),
 ( #33496, #9500, #38475 ),
 ( #4557, #3594, #28490 ),
 ( #44120, #60072, #39445 ),
 ( #14491, #24482, #4212 ),
 ( #43795, #59410, #33799 ),
 ( #50101, #53786, #48797 ),
 ( #3248, #18557, #44760 ),
 ( #64387, #13833, #54443 ),
 ( #8875, #44422, #29167 ),
 ( #24159, #34766, #14175 ),
 ( #34465, #26135, #856 ),
 ( #46412, #45415, #9843 ),
 ( #45107, #55743, #60385 ),
 ( #40423, #24826, #46102 ),
 ( #14809, #56744, #65369 ),
 ( #51743, #30453, #55404 ),
 ( #50750, #21126, #548 ),
 ( #41400, #5878, #10831 ),
 ( #19834, #20488, #40093 ),
 ( #35094, #30136, #50435 ),
 ( #4880, #40773, #60724 ),
 ( #25807, #25146, #45751 ),
 ( #10173, #20812, #35443 ),
 ( #65682, #31115, #5199 ),
 ( #56048, #25467, #41080 ),
 ( #61358, #20152, #15157 ),
 ( #215, #10490, #5542 ) ),
 .UNSPECIFIED., .F., .F., .F. ) 
 B_SPLINE_SURFACE_WITH_KNOTS ( ( 4, 2, 2, 2, 2, 2, 2, 2, 2, 2, 2, 2, 2, 2, 2, 2, 2, 2, 2, 2, 2, 2, 2, 2, 4 ),
 ( 3, 3 ),
 ( 0.06047842900482980344, 0.06367705432712369995, 0.06527636698827063433, 0.06687567964941758258, 0.06847499231056453084, 0.07007430497171146522, 0.07327293029400536173, 0.07647155561629924436, 0.07807086827744619262, 0.07967018093859312700, 0.08286880626088702351, 0.08446811892203395788, 0.08606743158318090614, 0.08926605690547478877, 0.09086536956662173703, 0.09246468222776868529, 0.09566330755006256792, 0.09726262021120951617, 0.09886193287235645055, 0.1020605581946503471, 0.1052591835169442297, 0.1068584961780911780, 0.1084578088392381123, 0.1100571215003850606, 0.1116564341615320088 ),
 ( 0.000000000000000000, 1.000000000000000000 ),
 .UNSPECIFIED. ) 
 GEOMETRIC_REPRESENTATION_ITEM ( )  RATIONAL_B_SPLINE_SURFACE ( (
 ( 1.000000000000000000, 0.4999999999999997224, 1.000000000000000000),
 ( 1.000000000000000000, 0.5048840838053595403, 1.000000000000000000),
 ( 1.000000000000000000, 0.5132072642500212778, 1.000000000000000000),
 ( 1.000000000000000000, 0.5290214861663710133, 1.000000000000000000),
 ( 1.000000000000000000, 0.5348648783786191796, 1.000000000000000000),
 ( 1.000000000000000000, 0.5473516051742142174, 1.000000000000000000),
 ( 1.000000000000000000, 0.5539126387906654347, 1.000000000000000000),
 ( 1.000000000000000000, 0.5674101295481297491, 1.000000000000000000),
 ( 1.000000000000000000, 0.5743474342084209372, 1.000000000000000000),
 ( 1.000000000000000000, 0.5883951384281623787, 1.000000000000000000),
 ( 1.000000000000000000, 0.5955302209472954633, 1.000000000000000000),
 ( 1.000000000000000000, 0.6167715304224314909, 1.000000000000000000),
 ( 1.000000000000000000, 0.6305661306848800995, 1.000000000000000000),
 ( 1.000000000000000000, 0.6565125894471021128, 1.000000000000000000),
 ( 1.000000000000000000, 0.6686743926052455267, 1.000000000000000000),
 ( 1.000000000000000000, 0.6851014456086111926, 1.000000000000000000),
 ( 1.000000000000000000, 0.6902475665164108376, 1.000000000000000000),
 ( 1.000000000000000000, 0.6997062435423183624, 1.000000000000000000),
 ( 1.000000000000000000, 0.7040363771866963161, 1.000000000000000000),
 ( 1.000000000000000000, 0.7157418617803246175, 1.000000000000000000),
 ( 1.000000000000000000, 0.7218341033858746147, 1.000000000000000000),
 ( 1.000000000000000000, 0.7280280015706425134, 1.000000000000000000),
 ( 1.000000000000000000, 0.7296036051598833172, 1.000000000000000000),
 ( 1.000000000000000000, 0.7316818214130011988, 1.000000000000000000),
 ( 1.000000000000000000, 0.7321927565543977501, 1.000000000000000000),
 ( 1.000000000000000000, 0.7321641879724063440, 1.000000000000000000),
 ( 1.000000000000000000, 0.7300624469251318915, 1.000000000000000000),
 ( 1.000000000000000000, 0.7238943330024291134, 1.000000000000000000),
 ( 1.000000000000000000, 0.7213359435419269827, 1.000000000000000000),
 ( 1.000000000000000000, 0.7152343487864535332, 1.000000000000000000),
 ( 1.000000000000000000, 0.7117056589943943079, 1.000000000000000000),
 ( 1.000000000000000000, 0.6999072021060611659, 1.000000000000000000),
 ( 1.000000000000000000, 0.6903911339383190793, 1.000000000000000000),
 ( 1.000000000000000000, 0.6741089150890113846, 1.000000000000000000),
 ( 1.000000000000000000, 0.6683461163769177649, 1.000000000000000000),
 ( 1.000000000000000000, 0.6562237482356456653, 1.000000000000000000),
 ( 1.000000000000000000, 0.6498375142660577364, 1.000000000000000000),
 ( 1.000000000000000000, 0.6302143011362419944, 1.000000000000000000),
 ( 1.000000000000000000, 0.6164540672887564021, 1.000000000000000000),
 ( 1.000000000000000000, 0.5885848209491307825, 1.000000000000000000),
 ( 1.000000000000000000, 0.5744580946949390254, 1.000000000000000000),
 ( 1.000000000000000000, 0.5540565490002423710, 1.000000000000000000),
 ( 1.000000000000000000, 0.5474350731751366217, 1.000000000000000000),
 ( 1.000000000000000000, 0.5350293539660311293, 1.000000000000000000),
 ( 1.000000000000000000, 0.5292092555093077522, 1.000000000000000000),
 ( 1.000000000000000000, 0.5186171472262492976, 1.000000000000000000),
 ( 1.000000000000000000, 0.5138445523878416576, 1.000000000000000000),
 ( 1.000000000000000000, 0.5056909436241932010, 1.000000000000000000),
 ( 1.000000000000000000, 0.5023956439952826925, 1.000000000000000000),
 ( 1.000000000000000000, 0.4999999999999995004, 1.000000000000000000) ) ) 
 REPRESENTATION_ITEM ( '' )  SURFACE ( )  );
#29927=CARTESIAN_POINT ( 'NONE',  ( 3.967932057708484894, -25.89885127696171097, 15.40358068932206237 ) ) ;
#29951=EDGE_CURVE ( 'NONE', #51562, #56931, #65539, .T. ) ;
#29959=VECTOR ( 'NONE', #45588, 1000.000000000000000 ) ;
#29961=CARTESIAN_POINT ( 'NONE',  ( -18.85528480568559928, -29.92804508438502253, -6.903306693652388581 ) ) ;
#29990=CARTESIAN_POINT ( 'NONE',  ( -11.13200843151506092, -27.92871652161695550, -13.87829993151233055 ) ) ;
#29995=ORIENTED_EDGE ( 'NONE', *, *, #28382, .F. ) ;
#30015=ORIENTED_EDGE ( 'NONE', *, *, #31015, .F. ) ;
#30036=CARTESIAN_POINT ( 'NONE',  ( 29.10325845542004686, -3.352553978523171274, 24.67444324980777992 ) ) ;
#30041=CARTESIAN_POINT ( 'NONE',  ( 15.82795513634610174, -34.24358411257765056, 7.361295665688344592 ) ) ;
#30066=CARTESIAN_POINT ( 'NONE',  ( -12.75996857643550797, -29.16082758670667019, 4.038023594093941959 ) ) ;
#30077=CARTESIAN_POINT ( 'NONE',  ( 16.79298069408870830, -34.48269025770200358, 5.249417709786182940 ) ) ;
#30136=CARTESIAN_POINT ( 'NONE',  ( 12.30974346995382973, -29.30943841933768823, -5.552318955346970064 ) ) ;
#30159=CARTESIAN_POINT ( 'NONE',  ( -25.00000000000000355, -30.00000000000000000, 5.000000000000000888 ) ) ;
#30180=LINE ( 'NONE', #50483, #29073 ) ;
#30205=CARTESIAN_POINT ( 'NONE',  ( 41.00000000000000711, -1.694065894508600678E-18, 0.000000000000000000 ) ) ;
#30220=CARTESIAN_POINT ( 'NONE',  ( -16.81801275797650419, -34.49999999999998579, 5.265606433706007117 ) ) ;
#30237=VERTEX_POINT ( 'NONE', #4999 ) ;
#30245=ADVANCED_FACE ( 'NONE', ( #45535 ), #49888, .T. ) ;
#30263=CARTESIAN_POINT ( 'NONE',  ( -16.02919692786943173, -28.24921752684736376, 10.30002093107130179 ) ) ;
#30286=CARTESIAN_POINT ( 'NONE',  ( -14.60253471108646472, -28.81751583403978145, 11.78204505887441655 ) ) ;
#30327=CARTESIAN_POINT ( 'NONE',  ( 4.513117160428445906, -30.90576903066049752, -14.85933548762053924 ) ) ;
#30355=DIRECTION ( 'NONE',  ( 0.000000000000000000, 0.000000000000000000, -1.000000000000000000 ) ) ;
#30368=DIRECTION ( 'NONE',  ( 0.000000000000000000, 1.000000000000000000, 0.000000000000000000 ) ) ;
#30372=CARTESIAN_POINT ( 'NONE',  ( -48.71973356879950501, -0.2586908456633208453, -8.066649094095314609 ) ) ;
#30375=CARTESIAN_POINT ( 'NONE',  ( 16.45009115226408269, -34.41505313721369674, 6.130398315943972776 ) ) ;
#30389=EDGE_LOOP ( 'NONE', ( #14557, #36654, #28289, #19800 ) ) ;
#30398=FACE_OUTER_BOUND ( 'NONE', #3768, .T. ) ;
#30409=CARTESIAN_POINT ( 'NONE',  ( 9.591596427418885185, -32.12122108032075118, 13.09346764506430283 ) ) ;
#30420=VERTEX_POINT ( 'NONE', #19133 ) ;
#30444=CARTESIAN_POINT ( 'NONE',  ( 15.45402751312076362, -34.86645063878552264, 6.224822664677306605 ) ) ;
#30453=CARTESIAN_POINT ( 'NONE',  ( 10.51584247049436449, -29.12274881419611106, -8.353506175201005135 ) ) ;
#30483=AXIS2_PLACEMENT_3D ( 'NONE', #24370, #30355, #25357 ) ;
#30503=DIRECTION ( 'NONE',  ( -1.000000000000000000, 0.000000000000000000, 0.000000000000000000 ) ) ;
#30517=CARTESIAN_POINT ( 'NONE',  ( -19.56743653832046803, -28.99999999999999645, -4.999999999999997335 ) ) ;
#30572=CARTESIAN_POINT ( 'NONE',  ( 15.64771680208055393, -28.15000396670248506, 10.66347899870800298 ) ) ;
#30574=DIRECTION ( 'NONE',  ( 1.000000000000000000, 0.000000000000000000, -0.000000000000000000 ) ) ;
#30592=CARTESIAN_POINT ( 'NONE',  ( -39.82259759989633352, -25.85751090193130253, -4.500000000000000000 ) ) ;
#30593=CARTESIAN_POINT ( 'NONE',  ( -17.14901781563218819, -29.51442629269803675, 9.398967198486925412 ) ) ;
#30614=CARTESIAN_POINT ( 'NONE',  ( 48.99862351417106510, -0.2022747408561471338, -1.593306619454940787 ) ) ;
#30632=CARTESIAN_POINT ( 'NONE',  ( 7.310206959903694290, -27.15910349781274391, -15.27822828334930705 ) ) ;
#30659=LINE ( 'NONE', #50971, #2178 ) ;
#30677=CARTESIAN_POINT ( 'NONE',  ( 49.99855491382518125, -0.0002949769214594301510, -1.660073069598956064 ) ) ;
#30678=CARTESIAN_POINT ( 'NONE',  ( 25.00000000000000355, -28.99999999999999645, 1.530808498934191521E-15 ) ) ;
#30685=ADVANCED_FACE ( 'NONE', ( #11760 ), #41213, .T. ) ;
#30719=CIRCLE ( 'NONE', #3139, 16.73205080756888563 ) ;
#30722=CARTESIAN_POINT ( 'NONE',  ( 12.39041149895467875, -29.91764912108355290, 8.475516454291387447 ) ) ;
#30794=AXIS2_PLACEMENT_3D ( 'NONE', #12542, #33505, #48167 ) ;
#30883=CARTESIAN_POINT ( 'NONE',  ( -14.30187556442842478, -30.10361765235437304, 4.782130246577438015 ) ) ;
#30890=ORIENTED_EDGE ( 'NONE', *, *, #25231, .T. ) ;
#30899=CARTESIAN_POINT ( 'NONE',  ( 19.56743653832047514, -28.99999999999999645, 4.999999999999997335 ) ) ;
#30927=CARTESIAN_POINT ( 'NONE',  ( 18.79103332550324623, -28.91360719445344785, -6.866334764117087985 ) ) ;
#30928=CARTESIAN_POINT ( 'NONE',  ( 19.24109636373442100, -29.98159021036885008, 5.977446804020324578 ) ) ;
#30952=CARTESIAN_POINT ( 'NONE',  ( 25.00000000000000711, -3.797884998337192286, -24.00000000000000000 ) ) ;
#30969=CARTESIAN_POINT ( 'NONE',  ( 16.45277491483739496, -34.41570230176855461, -6.124363151458832810 ) ) ;
#30971=ORIENTED_EDGE ( 'NONE', *, *, #55509, .T. ) ;
#30973=CARTESIAN_POINT ( 'NONE',  ( 0.000000000000000000, 244.9489742783177917, 24.99999999999999289 ) ) ;
#31015=EDGE_CURVE ( 'NONE', #18880, #14095, #50644, .T. ) ;
#31022=CARTESIAN_POINT ( 'NONE',  ( 49.59714883329486668, -0.08190040965285508290, 4.488761805454714704 ) ) ;
#31040=VERTEX_POINT ( 'NONE', #61912 ) ;
#31056=CARTESIAN_POINT ( 'NONE',  ( -0.8442279638247468521, -31.04755392045528950, 14.43184553624044852 ) ) ;
#31067=CARTESIAN_POINT ( 'NONE',  ( 14.42557999472123775, -30.05477271089676350, 4.241434648442734989 ) ) ;
#31115=CARTESIAN_POINT ( 'NONE',  ( 12.74086035833940045, -29.15670053398524431, -4.066541195106388784 ) ) ;
#31126=PRODUCT_DEFINITION ( 'UNKNOWN', '', #18669, #22623 ) ;
#31204=CIRCLE ( 'NONE', #2561, 4.500000000000000888 ) ;
#31214=DIRECTION ( 'NONE',  ( 1.000000000000000000, 0.000000000000000000, -0.000000000000000000 ) ) ;
#31239=CARTESIAN_POINT ( 'NONE',  ( -48.36589927958296187, -0.3279091627047597268, 5.494672883103054239 ) ) ;
#31271=LINE ( 'NONE', #27574, #23213 ) ;
#31272=CARTESIAN_POINT ( 'NONE',  ( 19.56743653832046803, -28.99999999999999645, -5.000000000000000888 ) ) ;
#31290=ORIENTED_EDGE ( 'NONE', *, *, #21302, .F. ) ;
#31291=EDGE_CURVE ( 'NONE', #37992, #32577, #24276, .T. ) ;
#31310=CARTESIAN_POINT ( 'NONE',  ( 19.27363075669124726, -29.98494805059728208, -5.891112176854690574 ) ) ;
#31319=DIRECTION ( 'NONE',  ( 0.000000000000000000, 1.000000000000000000, 0.000000000000000000 ) ) ;
#31341=EDGE_LOOP ( 'NONE', ( #34250, #27484, #4069, #1314 ) ) ;
#31352=CARTESIAN_POINT ( 'NONE',  ( 38.20713125073508110, -2.115151932665336076, 21.24219930640694898 ) ) ;
#31357=FACE_OUTER_BOUND ( 'NONE', #33504, .T. ) ;
#31387=CARTESIAN_POINT ( 'NONE',  ( 11.41243050843482187, -29.26822538582518263, 7.243948608349396245 ) ) ;
#31400=TOROIDAL_SURFACE ( 'NONE', #53681, 20.19615242270663558, 3.000000000000000000 ) ;
#31417=FACE_OUTER_BOUND ( 'NONE', #60815, .T. ) ;
#31436=CARTESIAN_POINT ( 'NONE',  ( 16.10065672031746331, -35.00000000000000711, 4.574893970807607957 ) ) ;
#31440=VERTEX_POINT ( 'NONE', #46541 ) ;
#31512=CARTESIAN_POINT ( 'NONE',  ( -33.80171706282990840, -2.756546641835186051, 23.41361577495085200 ) ) ;
#31549=CARTESIAN_POINT ( 'NONE',  ( -15.83540182711246835, -34.24586518154816872, -7.348477566591427923 ) ) ;
#31557=ORIENTED_EDGE ( 'NONE', *, *, #34653, .F. ) ;
#31565=VERTEX_POINT ( 'NONE', #28877 ) ;
#31566=LINE ( 'NONE', #61830, #37513 ) ;
#31580=CARTESIAN_POINT ( 'NONE',  ( -1.994964832131320920, -25.76766306558319286, -15.60102351411471666 ) ) ;
#31590=AXIS2_PLACEMENT_3D ( 'NONE', #46760, #62366, #41769 ) ;
#31602=CARTESIAN_POINT ( 'NONE',  ( 39.58329824467850244, -1.898237318462468792, -19.07749194152998129 ) ) ;
#31618=CARTESIAN_POINT ( 'NONE',  ( 14.19127861765052501, -30.11167671974727256, -5.095448428665124041 ) ) ;
#31655=FACE_OUTER_BOUND ( 'NONE', #52966, .T. ) ;
#31660=CARTESIAN_POINT ( 'NONE',  ( -25.00000000000000355, -9.999999999999998224, -4.999999999999999112 ) ) ;
#31692=CARTESIAN_POINT ( 'NONE',  ( 12.91449914267798960, -27.44768092100439461, 12.53791341943762916 ) ) ;
#31723=EDGE_CURVE ( 'NONE', #34331, #33819, #39171, .T. ) ;
#31734=CARTESIAN_POINT ( 'NONE',  ( -25.00000000000000355, -9.999999999999998224, -25.00000000000000000 ) ) ;
#31739=CARTESIAN_POINT ( 'NONE',  ( -41.00000000000000711, -25.30020925422648048, 3.022492086418944623 ) ) ;
#31742=CARTESIAN_POINT ( 'NONE',  ( 16.21117406328131949, -35.00000000000000000, 4.142385751841762165 ) ) ;
#31752=LINE ( 'NONE', #52722, #50912 ) ;
#31813=ORIENTED_EDGE ( 'NONE', *, *, #21302, .T. ) ;
#31824=CARTESIAN_POINT ( 'NONE',  ( -48.39008813825011401, -0.3233266992476376833, 8.863930066451535694 ) ) ;
#31833=CARTESIAN_POINT ( 'NONE',  ( -16.21117406328131594, -35.00000000000000000, -4.142385751841761277 ) ) ;
#31894=EDGE_LOOP ( 'NONE', ( #16478, #58541, #53773, #11877 ) ) ;
#31899=CARTESIAN_POINT ( 'NONE',  ( -0.9955874700083122697, -25.73414319850213516, -15.65071058219114342 ) ) ;
#31945=EDGE_LOOP ( 'NONE', ( #8017, #11056, #34560, #33932 ) ) ;
#31948=ORIENTED_EDGE ( 'NONE', *, *, #64334, .T. ) ;
#31959=VERTEX_POINT ( 'NONE', #48449 ) ;
#31996=CIRCLE ( 'NONE', #23525, 23.66025403784440329 ) ;
#32025=CARTESIAN_POINT ( 'NONE',  ( 9.730232070128172595, -26.74067542416307219, 13.98809302346541372 ) ) ;
#32033=CARTESIAN_POINT ( 'NONE',  ( 0.000000000000000000, -33.00000000000000000, 0.000000000000000000 ) ) ;
#32046=CARTESIAN_POINT ( 'NONE',  ( 0.000000000000000000, -30.00000000000000000, 0.000000000000000000 ) ) ;
#32068=CARTESIAN_POINT ( 'NONE',  ( -41.00000000000000711, -25.03188948156373783, 4.499999999999997335 ) ) ;
#32087=FACE_OUTER_BOUND ( 'NONE', #55441, .T. ) ;
#32110=AXIS2_PLACEMENT_3D ( 'NONE', #44530, #24262, #64807 ) ;
#32129=CARTESIAN_POINT ( 'NONE',  ( -25.00000000000000355, -9.999999999999998224, -5.000000000000000888 ) ) ;
#32155=CARTESIAN_POINT ( 'NONE',  ( -49.99855491382518835, -0.0002949769214475305985, 1.660073069598965390 ) ) ;
#32162=CARTESIAN_POINT ( 'NONE',  ( -17.92531974009704498, -28.72851451116432031, -8.222150688345376324 ) ) ;
#32194=DIRECTION ( 'NONE',  ( -0.9688695217174486674, 0.000000000000000000, -0.2475719085175094036 ) ) ;
#32197=CARTESIAN_POINT ( 'NONE',  ( -13.57005631242148347, -30.10739101144412544, -6.607437777791871802 ) ) ;
#32281=ORIENTED_EDGE ( 'NONE', *, *, #27463, .T. ) ;
#32309=LINE ( 'NONE', #52624, #52378 ) ;
#32321=CARTESIAN_POINT ( 'NONE',  ( 19.42209513767211604, -30.00000000000001066, -5.494601501491743534 ) ) ;
#32355=CARTESIAN_POINT ( 'NONE',  ( 3.413903065650966351, -31.27385512440588400, 14.18194743136197289 ) ) ;
#32402=CARTESIAN_POINT ( 'NONE',  ( 6.013273758146171488, -31.75304111243247007, 13.61309608153140793 ) ) ;
#32440=CARTESIAN_POINT ( 'NONE',  ( -46.85239813472878723, -0.6216812786252554623, 9.954194587011514272 ) ) ;
#32441=LINE ( 'NONE', #8490, #23510 ) ;
#32456=CARTESIAN_POINT ( 'NONE',  ( -37.25000000000000711, -27.41745588273159839, 3.011965929904363293 ) ) ;
#32458=LINE ( 'NONE', #21177, #12112 ) ;
#32486=CARTESIAN_POINT ( 'NONE',  ( -12.19463663866909187, -29.31670792731519626, -5.824636309907595511 ) ) ;
#32553=CARTESIAN_POINT ( 'NONE',  ( -19.56743653832047514, -28.99999999999999645, 5.000000000000000888 ) ) ;
#32577=VERTEX_POINT ( 'NONE', #56556 ) ;
#32588=DIRECTION ( 'NONE',  ( -0.9688695217174486674, 0.000000000000000000, -0.2475719085175094036 ) ) ;
#32603=DIRECTION ( 'NONE',  ( 0.000000000000000000, 0.000000000000000000, 1.000000000000000000 ) ) ;
#32615=ORIENTED_EDGE ( 'NONE', *, *, #26682, .T. ) ;
#32628=CARTESIAN_POINT ( 'NONE',  ( 7.964047368509766578, -27.27321649430781392, -15.08844977892397665 ) ) ;
#32639=EDGE_CURVE ( 'NONE', #38939, #38736, #65640, .T. ) ;
#32647=EDGE_CURVE ( 'NONE', #45854, #52466, #37627, .T. ) ;
#32663=CARTESIAN_POINT ( 'NONE',  ( 12.69762816655162574, -29.19309327991231839, 4.289906119467950418 ) ) ;
#32708=B_SPLINE_CURVE_WITH_KNOTS ( 'NONE', 3,
 ( #37276, #52275, #42929, #47927, #7690, #27975, #7028, #63209, #8031, #17991, #12334, #7340, #11675, #28298, #62876, #38253, #6716, #12649, #47285, #32933, #48283, #27625, #22990, #1725 ),
 .UNSPECIFIED., .F., .F.,
 ( 4, 2, 2, 2, 2, 2, 2, 2, 2, 2, 2, 4 ),
 ( 0.02095799966194190206, 0.02357897855711225260, 0.02619995745228260314, 0.02882093634745295369, 0.03013142579503812896, 0.03144191524262329729, 0.03406289413779364783, 0.03668387303296398450, 0.03799436248054915977, 0.03930485192813433504, 0.04061534137571949643, 0.04192583082330467170 ),
 .UNSPECIFIED. ) ;
#32724=VERTEX_POINT ( 'NONE', #36155 ) ;
#32726=DIRECTION ( 'NONE',  ( -0.000000000000000000, -0.000000000000000000, 1.000000000000000000 ) ) ;
#32753=CARTESIAN_POINT ( 'NONE',  ( -13.40508024068858894, -30.08919203116835206, 6.920461462857061541 ) ) ;
#32755=CARTESIAN_POINT ( 'NONE',  ( -48.84659035979349540, -0.2326159177122989752, -2.738175293146146050 ) ) ;
#32802=CARTESIAN_POINT ( 'NONE',  ( -50.00070814568297095, 0.0001445496031171917693, -0.7971761463862191421 ) ) ;
#32809=CARTESIAN_POINT ( 'NONE',  ( -14.06029564544070531, -34.40539544390912141, -8.431086515739542264 ) ) ;
#32842=CARTESIAN_POINT ( 'NONE',  ( -12.36714175812404015, -29.91041276695247575, -8.471522614803607354 ) ) ;
#32855=CARTESIAN_POINT ( 'NONE',  ( 19.56743653832047158, -33.00000000000000000, -5.000000000000017764 ) ) ;
#32861=ORIENTED_EDGE ( 'NONE', *, *, #48792, .T. ) ;
#32887=CARTESIAN_POINT ( 'NONE',  ( 4.563054428362612214, -30.91385115595551625, -14.84911024295102422 ) ) ;
#32894=CARTESIAN_POINT ( 'NONE',  ( -0.9215452301657053313, -30.54833844081648309, 15.29585404987972375 ) ) ;
#32903=CARTESIAN_POINT ( 'NONE',  ( 28.15855999187490966, -3.461419147680622199, 23.80441447217193840 ) ) ;
#32919=EDGE_CURVE ( 'NONE', #64219, #31959, #33620, .T. ) ;
#32933=CARTESIAN_POINT ( 'NONE',  ( 15.45402751311997847, -34.86645063878531658, -6.224822664678947959 ) ) ;
#32942=CARTESIAN_POINT ( 'NONE',  ( -1.327480008007509151E-11, -31.03649492335491544, -14.44372008463338908 ) ) ;
#32955=ADVANCED_FACE ( 'NONE', ( #58783 ), #60379, .T. ) ;
#32981=( BOUNDED_SURFACE ( )  B_SPLINE_SURFACE ( 3, 2, ( 
 ( #9782, #60324, #40358 ),
 ( #55995, #15742, #4496 ),
 ( #55343, #30066, #35698 ),
 ( #50035, #50696, #24763 ),
 ( #25092, #10767, #10432 ),
 ( #29726, #4825, #34710 ),
 ( #36020, #49707, #20095 ),
 ( #19782, #60659, #56319 ),
 ( #39724, #15097, #45043 ),
 ( #4154, #60016, #35375 ),
 ( #50378, #55683, #491 ),
 ( #5141, #24418, #14435 ),
 ( #45688, #5480, #55009 ),
 ( #65316, #10120, #9440 ),
 ( #40038, #25408, #147 ),
 ( #14752, #20428, #40705 ),
 ( #25748, #60997, #51019 ),
 ( #15431, #41025, #20756 ),
 ( #61308, #21064, #52344 ),
 ( #37687, #37347, #57983 ),
 ( #41345, #52003, #17411 ),
 ( #62285, #6447, #57316 ),
 ( #26726, #16740, #27057 ),
 ( #41686, #22378, #31056 ),
 ( #51688, #47021, #42643 ),
 ( #6130, #51366, #36699 ),
 ( #46675, #21755, #6783 ),
 ( #799, #1476, #61976 ),
 ( #7092, #42005, #32355 ),
 ( #46357, #62949, #16432 ),
 ( #56997, #61629, #47351 ),
 ( #11738, #26391, #1792 ),
 ( #16083, #37013, #26081 ),
 ( #32025, #22057, #42313 ),
 ( #62603, #17065, #57659 ),
 ( #12075, #1130, #21411 ),
 ( #11422, #52667, #5819 ),
 ( #31692, #36372, #27367 ),
 ( #2108, #47662, #56678 ),
 ( #11112, #31387, #59283 ),
 ( #37999, #58302, #8092 ),
 ( #63589, #13390, #13707 ),
 ( #63933, #12722, #28361 ),
 ( #13073, #33674, #27695 ),
 ( #38675, #18064, #53966 ),
 ( #38326, #32663, #18734 ),
 ( #58649, #33006, #53319 ),
 ( #8406, #7763, #28045 ),
 ( #49334, #18410, #48346 ),
 ( #3781, #28682, #48001 ) ),
 .UNSPECIFIED., .F., .F., .F. ) 
 B_SPLINE_SURFACE_WITH_KNOTS ( ( 4, 2, 2, 2, 2, 2, 2, 2, 2, 2, 2, 2, 2, 2, 2, 2, 2, 2, 2, 2, 2, 2, 2, 2, 4 ),
 ( 3, 3 ),
 ( 0.06047842900482980344, 0.06367705432712369995, 0.06527636698827063433, 0.06687567964941758258, 0.06847499231056453084, 0.07007430497171146522, 0.07327293029400536173, 0.07647155561629924436, 0.07807086827744619262, 0.07967018093859312700, 0.08286880626088702351, 0.08446811892203395788, 0.08606743158318090614, 0.08926605690547478877, 0.09086536956662173703, 0.09246468222776868529, 0.09566330755006256792, 0.09726262021120951617, 0.09886193287235645055, 0.1020605581946503471, 0.1052591835169442297, 0.1068584961780911780, 0.1084578088392381123, 0.1100571215003850606, 0.1116564341615320088 ),
 ( 0.000000000000000000, 1.000000000000000000 ),
 .UNSPECIFIED. ) 
 GEOMETRIC_REPRESENTATION_ITEM ( )  RATIONAL_B_SPLINE_SURFACE ( (
 ( 1.000000000000000000, 0.4999999999999997224, 1.000000000000000000),
 ( 1.000000000000000000, 0.5048840838053595403, 1.000000000000000000),
 ( 1.000000000000000000, 0.5132072642500212778, 1.000000000000000000),
 ( 1.000000000000000000, 0.5290214861663710133, 1.000000000000000000),
 ( 1.000000000000000000, 0.5348648783786191796, 1.000000000000000000),
 ( 1.000000000000000000, 0.5473516051742142174, 1.000000000000000000),
 ( 1.000000000000000000, 0.5539126387906654347, 1.000000000000000000),
 ( 1.000000000000000000, 0.5674101295481297491, 1.000000000000000000),
 ( 1.000000000000000000, 0.5743474342084209372, 1.000000000000000000),
 ( 1.000000000000000000, 0.5883951384281623787, 1.000000000000000000),
 ( 1.000000000000000000, 0.5955302209472954633, 1.000000000000000000),
 ( 1.000000000000000000, 0.6167715304224314909, 1.000000000000000000),
 ( 1.000000000000000000, 0.6305661306848800995, 1.000000000000000000),
 ( 1.000000000000000000, 0.6565125894471021128, 1.000000000000000000),
 ( 1.000000000000000000, 0.6686743926052455267, 1.000000000000000000),
 ( 1.000000000000000000, 0.6851014456086111926, 1.000000000000000000),
 ( 1.000000000000000000, 0.6902475665164108376, 1.000000000000000000),
 ( 1.000000000000000000, 0.6997062435423183624, 1.000000000000000000),
 ( 1.000000000000000000, 0.7040363771866963161, 1.000000000000000000),
 ( 1.000000000000000000, 0.7157418617803246175, 1.000000000000000000),
 ( 1.000000000000000000, 0.7218341033858746147, 1.000000000000000000),
 ( 1.000000000000000000, 0.7280280015706425134, 1.000000000000000000),
 ( 1.000000000000000000, 0.7296036051598833172, 1.000000000000000000),
 ( 1.000000000000000000, 0.7316818214130011988, 1.000000000000000000),
 ( 1.000000000000000000, 0.7321927565543977501, 1.000000000000000000),
 ( 1.000000000000000000, 0.7321641879724063440, 1.000000000000000000),
 ( 1.000000000000000000, 0.7300624469251318915, 1.000000000000000000),
 ( 1.000000000000000000, 0.7238943330024291134, 1.000000000000000000),
 ( 1.000000000000000000, 0.7213359435419269827, 1.000000000000000000),
 ( 1.000000000000000000, 0.7152343487864535332, 1.000000000000000000),
 ( 1.000000000000000000, 0.7117056589943943079, 1.000000000000000000),
 ( 1.000000000000000000, 0.6999072021060611659, 1.000000000000000000),
 ( 1.000000000000000000, 0.6903911339383190793, 1.000000000000000000),
 ( 1.000000000000000000, 0.6741089150890113846, 1.000000000000000000),
 ( 1.000000000000000000, 0.6683461163769177649, 1.000000000000000000),
 ( 1.000000000000000000, 0.6562237482356456653, 1.000000000000000000),
 ( 1.000000000000000000, 0.6498375142660577364, 1.000000000000000000),
 ( 1.000000000000000000, 0.6302143011362419944, 1.000000000000000000),
 ( 1.000000000000000000, 0.6164540672887564021, 1.000000000000000000),
 ( 1.000000000000000000, 0.5885848209491307825, 1.000000000000000000),
 ( 1.000000000000000000, 0.5744580946949390254, 1.000000000000000000),
 ( 1.000000000000000000, 0.5540565490002423710, 1.000000000000000000),
 ( 1.000000000000000000, 0.5474350731751366217, 1.000000000000000000),
 ( 1.000000000000000000, 0.5350293539660311293, 1.000000000000000000),
 ( 1.000000000000000000, 0.5292092555093077522, 1.000000000000000000),
 ( 1.000000000000000000, 0.5186171472262492976, 1.000000000000000000),
 ( 1.000000000000000000, 0.5138445523878416576, 1.000000000000000000),
 ( 1.000000000000000000, 0.5056909436241932010, 1.000000000000000000),
 ( 1.000000000000000000, 0.5023956439952826925, 1.000000000000000000),
 ( 1.000000000000000000, 0.4999999999999995004, 1.000000000000000000) ) ) 
 REPRESENTATION_ITEM ( '' )  SURFACE ( )  );
#32991=DIRECTION ( 'NONE',  ( 0.000000000000000000, -0.8660254037844380415, -0.5000000000000009992 ) ) ;
#33006=CARTESIAN_POINT ( 'NONE',  ( 12.74086035833940045, -29.15670053398430994, 4.066541195106272433 ) ) ;
#33052=CIRCLE ( 'NONE', #2273, 3.000000000000000444 ) ;
#33060=CARTESIAN_POINT ( 'NONE',  ( 4.340384785892905661, -31.41030204081990362, 14.02840248442622695 ) ) ;
#33087=CYLINDRICAL_SURFACE ( 'NONE', #64803, 24.00000000000000000 ) ;
#33101=CARTESIAN_POINT ( 'NONE',  ( -12.92674250727408669, -33.23908083898133015, 10.84893670414254530 ) ) ;
#33103=CARTESIAN_POINT ( 'NONE',  ( -44.04183182023682974, -1.142706581721706138, 14.69327751537514715 ) ) ;
#33132=CARTESIAN_POINT ( 'NONE',  ( -25.00000000000000355, -28.99999999999999645, 5.000000000000000888 ) ) ;
#33154=CARTESIAN_POINT ( 'NONE',  ( -13.72965000697191584, -27.65230582893893896, -12.05355732046426809 ) ) ;
#33165=VERTEX_POINT ( 'NONE', #33648 ) ;
#33178=EDGE_LOOP ( 'NONE', ( #37393, #50218, #36723, #52552 ) ) ;
#33240=CARTESIAN_POINT ( 'NONE',  ( 0.000000000000000000, -30.00000000000000000, 0.000000000000000000 ) ) ;
#33253=CARTESIAN_POINT ( 'NONE',  ( 32.73308617475132820, -2.903166307960730830, 22.77405829473931576 ) ) ;
#33317=CARTESIAN_POINT ( 'NONE',  ( 18.81741048081454082, -29.91393404465042138, -6.911695701493956179 ) ) ;
#33334=DIRECTION ( 'NONE',  ( -1.000000000000000000, -0.000000000000000000, -0.000000000000000000 ) ) ;
#33341=CARTESIAN_POINT ( 'NONE',  ( -37.25000000000000711, -20.00000000000000000, 2.449293598294706907E-15 ) ) ;
#33343=VERTEX_POINT ( 'NONE', #4047 ) ;
#33441=CARTESIAN_POINT ( 'NONE',  ( -0.5153900578009965594, -26.55329395651783031, 16.22445808467987050 ) ) ;
#33445=CARTESIAN_POINT ( 'NONE',  ( -39.62372872010315916, -1.894461972532858196, -19.09391518418255629 ) ) ;
#33496=CARTESIAN_POINT ( 'NONE',  ( -0.8442279638247468521, -31.04755392045528950, -14.43184553624044852 ) ) ;
#33504=EDGE_LOOP ( 'NONE', ( #26373, #24936 ) ) ;
#33505=DIRECTION ( 'NONE',  ( 0.2475719085175094314, 0.000000000000000000, -0.9688695217174487784 ) ) ;
#33520=VERTEX_POINT ( 'NONE', #37900 ) ;
#33543=DIRECTION ( 'NONE',  ( 0.000000000000000000, 0.000000000000000000, 1.000000000000000000 ) ) ;
#33561=EDGE_LOOP ( 'NONE', ( #48235, #59968, #9370, #12675 ) ) ;
#33603=CIRCLE ( 'NONE', #47426, 4.500000000000000888 ) ;
#33616=CARTESIAN_POINT ( 'NONE',  ( -17.71439793346020153, -28.67846309484135503, 8.502197385450015688 ) ) ;
#33620=B_SPLINE_CURVE_WITH_KNOTS ( 'NONE', 3,
 ( #27501, #16876, #37147, #36831, #22867, #47161, #31512, #47796, #22532, #57129, #58436, #6261, #52478, #58109, #12521, #51813, #11557, #37486, #17546, #31824, #6591, #26857, #27184, #1610, #27841, #21881, #32155, #32802, #19754, #29697, #50352, #54980, #2914, #10091, #30372, #50006, #9408, #40011, #53455, #28175, #60298, #65593, #50667, #114, #60626, #12864, #64064, #25377, #28480, #63718, #45333, #5111, #45660, #20394 ),
 .UNSPECIFIED., .F., .F.,
 ( 4, 2, 2, 2, 2, 2, 2, 2, 2, 2, 2, 2, 2, 2, 2, 2, 2, 2, 2, 2, 2, 2, 2, 2, 2, 2, 4 ),
 ( 0.000000000000000000, 0.004909564951003677659, 0.007364347426505511718, 0.009819129902007346644, 0.01472869485301101650, 0.01718347732851285489, 0.01963825980401469329, 0.02454782475501837702, 0.02700260723052021195, 0.02945738970602204687, 0.03191217218152388180, 0.03313956341927479926, 0.03436695465702571672, 0.03927651960802939352, 0.04173130208353122844, 0.04295869332128215284, 0.04418608455903307031, 0.04909564951003672628, 0.05155043198553856121, 0.05400521446104038920, 0.05891477941204405211, 0.06382434436304770808, 0.06627912683854954301, 0.06873390931405137794, 0.07364347426505504779, 0.07609825674055689659, 0.07855303921605873152 ),
 .UNSPECIFIED. ) ;
#33648=CARTESIAN_POINT ( 'NONE',  ( 25.00000000000000355, -9.999999999999998224, 24.00000000000000000 ) ) ;
#33660=CARTESIAN_POINT ( 'NONE',  ( 39.82259759989631931, -25.85751090193130608, -4.500000000000000000 ) ) ;
#33674=CARTESIAN_POINT ( 'NONE',  ( 12.50310467286144167, -29.27802453453052323, 5.021082754746532650 ) ) ;
#33682=CIRCLE ( 'NONE', #50686, 3.000000000000001332 ) ;
#33748=CARTESIAN_POINT ( 'NONE',  ( -7.529925403075611534, -31.54078451673377614, 13.99923386364726063 ) ) ;
#33765=CARTESIAN_POINT ( 'NONE',  ( -41.00000000000000711, -1.694065894508600678E-18, 0.000000000000000000 ) ) ;
#33777=LINE ( 'NONE', #33132, #48930 ) ;
#33795=CIRCLE ( 'NONE', #8327, 1.500000000000000222 ) ;
#33799=CARTESIAN_POINT ( 'NONE',  ( 3.702144525957873356, -25.87585389521097312, -15.43847573974272613 ) ) ;
#33819=VERTEX_POINT ( 'NONE', #21561 ) ;
#33824=( NAMED_UNIT ( * ) SI_UNIT ( $, .STERADIAN. ) SOLID_ANGLE_UNIT ( ) );
#33869=ADVANCED_FACE ( 'NONE', ( #48154 ), #29891, .T. ) ;
#33875=EDGE_CURVE ( 'NONE', #60939, #26603, #31752, .T. ) ;
#33886=AXIS2_PLACEMENT_3D ( 'NONE', #64440, #53526, #39176 ) ;
#33890=CARTESIAN_POINT ( 'NONE',  ( -9.668839327557112284, -32.14098936784372285, 13.07247934321766181 ) ) ;
#33906=CIRCLE ( 'NONE', #57280, 3.000000000000000444 ) ;
#33932=ORIENTED_EDGE ( 'NONE', *, *, #53860, .T. ) ;
#33959=CARTESIAN_POINT ( 'NONE',  ( -16.81808179455697427, -29.42526233323303941, -9.774508714121761699 ) ) ;
#34075=CARTESIAN_POINT ( 'NONE',  ( -4.505835087371258041, -30.89562805149345337, 14.87534964460356512 ) ) ;
#34081=ORIENTED_EDGE ( 'NONE', *, *, #27794, .F. ) ;
#34091=DIRECTION ( 'NONE',  ( -0.9688695217174487784, 0.000000000000000000, 0.2475719085175093481 ) ) ;
#34114=CIRCLE ( 'NONE', #42605, 16.19615242270663558 ) ;
#34118=CARTESIAN_POINT ( 'NONE',  ( 37.25000000000000711, -1.694065894508600678E-18, 0.000000000000000000 ) ) ;
#34125=CARTESIAN_POINT ( 'NONE',  ( -12.89187373143239945, -27.44222185127960145, -12.55025375818352629 ) ) ;
#34167=EDGE_LOOP ( 'NONE', ( #5398, #14739, #53796, #42173 ) ) ;
#34207=CARTESIAN_POINT ( 'NONE',  ( 16.93394556191327283, -34.50000000000001421, -4.811904876957583177 ) ) ;
#34218=CARTESIAN_POINT ( 'NONE',  ( -15.84367078531945516, -34.24835312396420051, 7.333865081865427626 ) ) ;
#34247=DIRECTION ( 'NONE',  ( 0.000000000000000000, 1.000000000000000000, 0.000000000000000000 ) ) ;
#34250=ORIENTED_EDGE ( 'NONE', *, *, #59041, .F. ) ;
#34253=ORIENTED_EDGE ( 'NONE', *, *, #25939, .F. ) ;
#34261=CARTESIAN_POINT ( 'NONE',  ( -0.9215452301825294290, -30.54833844081706928, -15.29585404987903452 ) ) ;
#34293=DIRECTION ( 'NONE',  ( 0.000000000000000000, 0.000000000000000000, 1.000000000000000000 ) ) ;
#34297=DIRECTION ( 'NONE',  ( -1.000000000000000000, 0.000000000000000000, 0.000000000000000000 ) ) ;
#34328=CARTESIAN_POINT ( 'NONE',  ( 1.819964709950166126, -30.58339181399412254, -15.25524951094132398 ) ) ;
#34331=VERTEX_POINT ( 'NONE', #14271 ) ;
#34360=EDGE_CURVE ( 'NONE', #12741, #39511, #19095, .T. ) ;
#34364=CARTESIAN_POINT ( 'NONE',  ( 16.21117406328131594, -35.00000000000000000, -4.142385751841773711 ) ) ;
#34414=CONICAL_SURFACE ( 'NONE', #42904, 14.13397459621556251, 0.5235987755983000369 ) ;
#34418=CARTESIAN_POINT ( 'NONE',  ( -3.619268891295738477, -30.76314776371165749, 15.03790153758943404 ) ) ;
#34449=CARTESIAN_POINT ( 'NONE',  ( 37.25000000000000711, 1.820029539775944174E-16, -1.500000000000000222 ) ) ;
#34465=CARTESIAN_POINT ( 'NONE',  ( 7.919433923537877895, -32.26502814485947823, -12.92562328492908286 ) ) ;
#34507=DIRECTION ( 'NONE',  ( 0.000000000000000000, 1.000000000000000000, 0.000000000000000000 ) ) ;
#34532=ADVANCED_FACE ( 'NONE', ( #52158 ), #56481, .F. ) ;
#34544=CARTESIAN_POINT ( 'NONE',  ( -15.09490394635158772, -34.00569493827280354, 8.490101771333646852 ) ) ;
#34549=VERTEX_POINT ( 'NONE', #50841 ) ;
#34560=ORIENTED_EDGE ( 'NONE', *, *, #26682, .F. ) ;
#34591=EDGE_CURVE ( 'NONE', #23145, #65150, #46765, .T. ) ;
#34612=CYLINDRICAL_SURFACE ( 'NONE', #6363, 24.00000000000000000 ) ;
#34639=CARTESIAN_POINT ( 'NONE',  ( -14.91771861688873635, -28.90354855594910433, -11.53870211790012412 ) ) ;
#34653=EDGE_CURVE ( 'NONE', #939, #34331, #1108, .T. ) ;
#34681=CARTESIAN_POINT ( 'NONE',  ( 44.83472798829955508, -0.9996270273486139724, -15.30615170800020586 ) ) ;
#34700=EDGE_LOOP ( 'NONE', ( #19285, #53398, #54938, #61955 ) ) ;
#34710=CARTESIAN_POINT ( 'NONE',  ( -14.32520573871325631, -34.50054679313745964, 8.085438606780256166 ) ) ;
#34721=CARTESIAN_POINT ( 'NONE',  ( 10.72528909898963789, -29.54774166152794734, 10.19639468772756530 ) ) ;
#34751=CARTESIAN_POINT ( 'NONE',  ( 0.000000000000000000, 244.9489742783177917, 23.99999999999999289 ) ) ;
#34766=CARTESIAN_POINT ( 'NONE',  ( 6.676753782886446942, -28.39896155677452683, -11.13103273143453720 ) ) ;
#34776=DIRECTION ( 'NONE',  ( 0.000000000000000000, 0.000000000000000000, 1.000000000000000000 ) ) ;
#34792=CARTESIAN_POINT ( 'NONE',  ( 0.000000000000000000, -45.00000000000000000, 0.000000000000000000 ) ) ;
#34845=DIRECTION ( 'NONE',  ( 0.000000000000000000, 0.000000000000000000, 1.000000000000000000 ) ) ;
#34846=CARTESIAN_POINT ( 'NONE',  ( -13.30196514322326529, -33.37310655729285003, 10.51054543287779097 ) ) ;
#34878=CARTESIAN_POINT ( 'NONE',  ( 0.000000000000000000, -33.00000000000000000, 0.000000000000000000 ) ) ;
#34893=CARTESIAN_POINT ( 'NONE',  ( -5.894163417187625598, -31.16155000483812998, -14.52685451767917080 ) ) ;
#34941=VERTEX_POINT ( 'NONE', #17143 ) ;
#34956=CARTESIAN_POINT ( 'NONE',  ( -4.505835087370986258, -30.89562805149607172, -14.87534964460527753 ) ) ;
#34960=DIRECTION ( 'NONE',  ( 1.000000000000000000, 0.000000000000000000, 0.000000000000000000 ) ) ;
#34964=DIRECTION ( 'NONE',  ( 1.000000000000000000, -0.000000000000000000, -0.000000000000000000 ) ) ;
#34984=AXIS2_PLACEMENT_3D ( 'NONE', #1316, #27540, #17588 ) ;
#34998=CARTESIAN_POINT ( 'NONE',  ( 40.23304019309009760, -1.796181362175405249, 19.88949158386753524 ) ) ;
#35003=CARTESIAN_POINT ( 'NONE',  ( 4.563054428376214666, -30.91385115595774735, 14.84911024294817850 ) ) ;
#35042=CARTESIAN_POINT ( 'NONE',  ( 6.263846918918718920, -28.63916073140924112, 12.80708683763934808 ) ) ;
#35047=CARTESIAN_POINT ( 'NONE',  ( 19.56743653832047514, -33.00000000000000000, 5.000000000000001776 ) ) ;
#35051=ADVANCED_FACE ( 'NONE', ( #31655 ), #14884, .F. ) ;
#35062=AXIS2_PLACEMENT_3D ( 'NONE', #8159, #58727, #2865 ) ;
#35089=CARTESIAN_POINT ( 'NONE',  ( -1.327480008007509151E-11, -31.03649492335491544, -14.44372008463338908 ) ) ;
#35094=CARTESIAN_POINT ( 'NONE',  ( 14.32183389819027930, -34.49933334076765590, -8.089813643623637418 ) ) ;
#35186=ADVANCED_FACE ( 'NONE', ( #5935, #1256 ), #21536, .F. ) ;
#35193=ORIENTED_EDGE ( 'NONE', *, *, #50249, .T. ) ;
#35217=ORIENTED_EDGE ( 'NONE', *, *, #18269, .T. ) ;
#35233=CARTESIAN_POINT ( 'NONE',  ( -1.994964832131321808, -25.76766306558318220, 15.60102351411471666 ) ) ;
#35252=EDGE_CURVE ( 'NONE', #659, #11368, #33777, .T. ) ;
#35256=CARTESIAN_POINT ( 'NONE',  ( -17.77323790556441452, -29.67638950762373895, 8.606028548248493948 ) ) ;
#35297=CARTESIAN_POINT ( 'NONE',  ( -4.228765754682466849, -26.75056327283501290, -15.92880586833495649 ) ) ;
#35299=DIRECTION ( 'NONE',  ( 0.2475719085175094591, 6.192417051524157726E-18, -0.9688695217174487784 ) ) ;
#35307=CARTESIAN_POINT ( 'NONE',  ( -2.195494320936263843, -31.13300424730153892, 14.33890400575774215 ) ) ;
#35313=FACE_OUTER_BOUND ( 'NONE', #42240, .T. ) ;
#35342=EDGE_CURVE ( 'NONE', #15192, #37781, #12507, .T. ) ;
#35350=CARTESIAN_POINT ( 'NONE',  ( 16.78995969943036570, -34.48221411999240615, 5.258039666742008400 ) ) ;
#35369=ORIENTED_EDGE ( 'NONE', *, *, #28100, .F. ) ;
#35375=CARTESIAN_POINT ( 'NONE',  ( -12.58725039716645000, -33.86007533429943095, 10.00564543523592320 ) ) ;
#35387=CARTESIAN_POINT ( 'NONE',  ( 13.74768401152558894, -28.58623978001741861, 12.41178146356747192 ) ) ;
#35437=CARTESIAN_POINT ( 'NONE',  ( -9.179144435738862740, -32.64956785250165439, -12.36195000407440148 ) ) ;
#35443=CARTESIAN_POINT ( 'NONE',  ( 18.66975156949834513, -28.88996333714986875, -7.079161351701957372 ) ) ;
#35570=CARTESIAN_POINT ( 'NONE',  ( -10.65145977119705201, -26.92745566885138686, 13.64141904900985836 ) ) ;
#35571=DIRECTION ( 'NONE',  ( 0.000000000000000000, 0.000000000000000000, 1.000000000000000000 ) ) ;
#35590=DIRECTION ( 'NONE',  ( 0.000000000000000000, 0.000000000000000000, -1.000000000000000000 ) ) ;
#35591=CARTESIAN_POINT ( 'NONE',  ( -10.65145977119704845, -26.92745566885138331, -13.64141904900985836 ) ) ;
#35592=CARTESIAN_POINT ( 'NONE',  ( -4.047649113456393444, -26.73415408998407372, 15.95376587162193260 ) ) ;
#35614=CARTESIAN_POINT ( 'NONE',  ( 33.44920912455760487, -2.804301875032225944, -22.47723755754418562 ) ) ;
#35623=CARTESIAN_POINT ( 'NONE',  ( 25.00000000000000711, -3.797884998337192286, -25.00000000000000000 ) ) ;
#35630=CARTESIAN_POINT ( 'NONE',  ( -3.619268891295734480, -30.76314776371165749, -15.03790153758943582 ) ) ;
#35639=CARTESIAN_POINT ( 'NONE',  ( -15.99047871552748390, -35.00000000000000000, 5.006074194136941991 ) ) ;
#35643=PLANE ( 'NONE',  #5356 ) ;
#35671=CARTESIAN_POINT ( 'NONE',  ( 49.96127604611442052, -0.007915161567782847199, 1.618137530678326552 ) ) ;
#35676=CARTESIAN_POINT ( 'NONE',  ( 5.011577697835214451, -30.99110506585922664, 14.75067033891186696 ) ) ;
#35693=DIRECTION ( 'NONE',  ( 0.000000000000000000, -1.000000000000000000, 0.000000000000000000 ) ) ;
#35698=CARTESIAN_POINT ( 'NONE',  ( -15.66605021877826331, -34.92947327577397942, 5.825441821991796942 ) ) ;
#35709=CARTESIAN_POINT ( 'NONE',  ( 19.43600551875679017, -29.99999999999999645, 5.447264023289953627 ) ) ;
#35730=ORIENTED_EDGE ( 'NONE', *, *, #38364, .F. ) ;
#35763=DIRECTION ( 'NONE',  ( 0.000000000000000000, 0.000000000000000000, 1.000000000000000000 ) ) ;
#35780=EDGE_LOOP ( 'NONE', ( #22768, #4905, #59184, #24002 ) ) ;
#35818=CARTESIAN_POINT ( 'NONE',  ( 25.00000000000000355, -3.797884998337192286, 23.99999999999999289 ) ) ;
#35863=ORIENTED_EDGE ( 'NONE', *, *, #5223, .F. ) ;
#35900=CARTESIAN_POINT ( 'NONE',  ( -1.009501604528838081, -26.56249173023641674, 16.21092882686939518 ) ) ;
#35938=CARTESIAN_POINT ( 'NONE',  ( 11.12775972613913211, -27.93149659178525823, -13.86083901436714427 ) ) ;
#35957=ORIENTED_EDGE ( 'NONE', *, *, #19492, .F. ) ;
#36013=CARTESIAN_POINT ( 'NONE',  ( -25.00000000000000355, -9.999999999999998224, 1.530808498934191521E-15 ) ) ;
#36020=CARTESIAN_POINT ( 'NONE',  ( -17.03240540343445630, -28.50880493221823286, 9.306303259374256953 ) ) ;
#36021=B_SPLINE_CURVE_WITH_KNOTS ( 'NONE', 3,
 ( #49759, #50096, #51080, #542, #45100, #24477, #15151, #19509, #25802, #20147, #19829, #40088, #29779, #35437, #41075, #20483, #46095, #65035, #60067, #4551, #65364, #60377, #25141, #20807, #14803, #35089 ),
 .UNSPECIFIED., .F., .F.,
 ( 4, 2, 2, 2, 2, 2, 2, 2, 2, 2, 2, 2, 4 ),
 ( 0.000000000000000000, 0.002619749957742739058, 0.003929624936614107070, 0.005239499915485476382, 0.006549374894356846562, 0.007859249873228217609, 0.01047899983097095103, 0.01309874978871368618, 0.01440862476758505810, 0.01571849974645642828, 0.01833824970419916517, 0.01964812468307053708, 0.02095799966194190206 ),
 .UNSPECIFIED. ) ;
#36033=CARTESIAN_POINT ( 'NONE',  ( 7.125164966885773055, -31.43290117443686071, 14.16047883281854425 ) ) ;
#36034=ADVANCED_FACE ( 'NONE', ( #25880 ), #285, .F. ) ;
#36071=AXIS2_PLACEMENT_3D ( 'NONE', #44883, #34247, #8987 ) ;
#36134=DIRECTION ( 'NONE',  ( 0.000000000000000000, 0.000000000000000000, -1.000000000000000000 ) ) ;
#36155=CARTESIAN_POINT ( 'NONE',  ( 0.000000000000000000, -45.00000000000000000, -22.50555349946515804 ) ) ;
#36194=CARTESIAN_POINT ( 'NONE',  ( -17.03240540343445630, -29.48295256022971955, 9.532950799341300296 ) ) ;
#36200=CARTESIAN_POINT ( 'NONE',  ( -28.93866847389638153, -3.371687389997700901, -23.68754010782029340 ) ) ;
#36202=EDGE_LOOP ( 'NONE', ( #6138, #10435, #8075, #51868, #52936, #10501 ) ) ;
#36211=CARTESIAN_POINT ( 'NONE',  ( -4.968020780095185884, -25.99038707641917156, 15.26464785194326979 ) ) ;
#36236=CARTESIAN_POINT ( 'NONE',  ( 0.000000000000000000, -35.00000000000000000, 0.000000000000000000 ) ) ;
#36266=CARTESIAN_POINT ( 'NONE',  ( 22.00000000000000711, -20.00000000000000000, 2.449293598294706907E-15 ) ) ;
#36278=CARTESIAN_POINT ( 'NONE',  ( 37.25000000000000711, -27.53407839942726909, 1.504154570186529094 ) ) ;
#36283=CARTESIAN_POINT ( 'NONE',  ( 12.91449914267889731, -28.36597991684663000, -12.93464570467139119 ) ) ;
#36329=ORIENTED_EDGE ( 'NONE', *, *, #34653, .T. ) ;
#36331=VECTOR ( 'NONE', #48215, 1000.000000000000000 ) ;
#36372=CARTESIAN_POINT ( 'NONE',  ( 9.989421171649008002, -29.02163280020532099, 8.890648868200056398 ) ) ;
#36423=CARTESIAN_POINT ( 'NONE',  ( 9.160076034430323588, -32.64719971958564315, 12.35384511440123134 ) ) ;
#36430=PLANE ( 'NONE',  #50229 ) ;
#36447=CARTESIAN_POINT ( 'NONE',  ( 19.56743653832047158, -33.00000000000000000, 5.000000000000007994 ) ) ;
#36495=EDGE_LOOP ( 'NONE', ( #49909, #15946, #55497, #20476 ) ) ;
#36525=CIRCLE ( 'NONE', #45019, 1.500000000000000444 ) ;
#36527=ORIENTED_EDGE ( 'NONE', *, *, #39849, .F. ) ;
#36544=CARTESIAN_POINT ( 'NONE',  ( 41.00000000000000711, -25.49198847189177997, 0.7539676769129244338 ) ) ;
#36550=CARTESIAN_POINT ( 'NONE',  ( -15.59741926309910021, -34.17135967094492344, -7.744809993483719346 ) ) ;
#36554=CARTESIAN_POINT ( 'NONE',  ( 37.25000000000000711, -1.694065894508793271E-18, 4.500000000000001776 ) ) ;
#36585=CARTESIAN_POINT ( 'NONE',  ( 17.69916095700584080, -28.67478364583445583, -8.521665482016093307 ) ) ;
#36586=CARTESIAN_POINT ( 'NONE',  ( 9.836964722002420558, -27.64452029744604999, 14.41904541651817340 ) ) ;
#36607=CARTESIAN_POINT ( 'NONE',  ( 45.77739315166651579, -0.8244463642989235952, 12.03838484699754652 ) ) ;
#36618=CARTESIAN_POINT ( 'NONE',  ( 37.25000000000000711, -27.21021009056489248, -4.500000000000000888 ) ) ;
#36623=CARTESIAN_POINT ( 'NONE',  ( 10.72528909898949401, -29.54774166153168835, -10.19639468772673219 ) ) ;
#36633=CARTESIAN_POINT ( 'NONE',  ( -12.63451720667688072, -33.87771254755728734, 9.962109630954579131 ) ) ;
#36654=ORIENTED_EDGE ( 'NONE', *, *, #11958, .T. ) ;
#36699=CARTESIAN_POINT ( 'NONE',  ( 0.8665813290829081916, -31.03691730605172694, 14.44326482629603881 ) ) ;
#36723=ORIENTED_EDGE ( 'NONE', *, *, #52524, .T. ) ;
#36726=DIRECTION ( 'NONE',  ( -0.000000000000000000, -1.000000000000000000, -0.000000000000000000 ) ) ;
#36802=CARTESIAN_POINT ( 'NONE',  ( 1.836970198721029589E-15, -30.00000000000000000, 15.00000000000000000 ) ) ;
#36821=EDGE_CURVE ( 'NONE', #14095, #60939, #21467, .T. ) ;
#36831=CARTESIAN_POINT ( 'NONE',  ( -30.66651853351973145, -3.164325622109353642, 24.36290982288814888 ) ) ;
#36866=VECTOR ( 'NONE', #19792, 1000.000000000000000 ) ;
#36902=CARTESIAN_POINT ( 'NONE',  ( 18.54281746013980481, -28.86505449477129659, -7.298814700743937678 ) ) ;
#36922=CARTESIAN_POINT ( 'NONE',  ( 44.06649112733599338, -1.138262461040735474, 14.66001971352460309 ) ) ;
#36939=CARTESIAN_POINT ( 'NONE',  ( 19.56743653832047869, -29.99999999999999645, -4.999999999999984013 ) ) ;
#36950=DIRECTION ( 'NONE',  ( 0.000000000000000000, 1.000000000000000000, 0.000000000000000000 ) ) ;
#37013=CARTESIAN_POINT ( 'NONE',  ( 6.676753782886446942, -28.39896155677633516, 11.13103273143544314 ) ) ;
#37062=CARTESIAN_POINT ( 'NONE',  ( 3.474089039520120270, -31.27092243478756117, 14.18576039181575688 ) ) ;
#37076=ORIENTED_EDGE ( 'NONE', *, *, #13546, .T. ) ;
#37087=CARTESIAN_POINT ( 'NONE',  ( 22.00000000000000711, -20.00000000000000000, -1.499999999999998002 ) ) ;
#37118=CARTESIAN_POINT ( 'NONE',  ( 0.000000000000000000, -45.00000000000000000, 0.000000000000000000 ) ) ;
#37147=CARTESIAN_POINT ( 'NONE',  ( -28.27451930523357149, -3.452175767011101737, 24.83788945613662236 ) ) ;
#37152=CARTESIAN_POINT ( 'NONE',  ( -19.30028080049353179, -29.00000000000000000, -5.863682654924961213 ) ) ;
#37184=CARTESIAN_POINT ( 'NONE',  ( -14.43403921783542998, -30.05772736394682454, -4.235651140256554648 ) ) ;
#37212=EDGE_CURVE ( 'NONE', #52741, #33343, #5473, .T. ) ;
#37219=CARTESIAN_POINT ( 'NONE',  ( 12.54355452190763920, -28.27128177340750526, 13.14909765253697849 ) ) ;
#37233=VERTEX_POINT ( 'NONE', #54094 ) ;
#37245=ORIENTED_EDGE ( 'NONE', *, *, #8280, .F. ) ;
#37248=DIRECTION ( 'NONE',  ( 0.000000000000000000, 1.000000000000000000, 0.000000000000000000 ) ) ;
#37276=CARTESIAN_POINT ( 'NONE',  ( -1.327480008007509151E-11, -31.03649492335491544, -14.44372008463338908 ) ) ;
#37298=AXIS2_PLACEMENT_3D ( 'NONE', #34118, #54437, #7553 ) ;
#37311=EDGE_CURVE ( 'NONE', #33819, #53510, #36021, .T. ) ;
#37347=CARTESIAN_POINT ( 'NONE',  ( -4.291397156012838110, -28.05769852054401881, 12.02237517917411047 ) ) ;
#37350=DIRECTION ( 'NONE',  ( 0.000000000000000000, 0.000000000000000000, 1.000000000000000000 ) ) ;
#37388=CIRCLE ( 'NONE', #3444, 3.999999999999999556 ) ;
#37391=LINE ( 'NONE', #31734, #41568 ) ;
#37393=ORIENTED_EDGE ( 'NONE', *, *, #32639, .F. ) ;
#37429=VECTOR ( 'NONE', #33334, 1000.000000000000000 ) ;
#37439=CARTESIAN_POINT ( 'NONE',  ( -48.68114316863543678, -0.2655233219083077412, -3.919294168552598379 ) ) ;
#37456=CARTESIAN_POINT ( 'NONE',  ( -37.25000000000001421, -27.44817602132958356, -3.024649682742615919 ) ) ;
#37484=AXIS2_PLACEMENT_3D ( 'NONE', #34792, #40119, #50776 ) ;
#37486=CARTESIAN_POINT ( 'NONE',  ( -47.41189015808931373, -0.5144011408980343480, 11.10762064040664221 ) ) ;
#37493=CARTESIAN_POINT ( 'NONE',  ( -18.91767133624980701, -28.94173879345719058, -6.680047468371234309 ) ) ;
#37513=VECTOR ( 'NONE', #11937, 1000.000000000000000 ) ;
#37528=CARTESIAN_POINT ( 'NONE',  ( -14.21898193534930144, -33.70038524408754910, -9.575031237889035651 ) ) ;
#37627=B_SPLINE_CURVE_WITH_KNOTS ( 'NONE', 3,
 ( #16960, #12954, #53547, #52564, #12608, #32887, #53198, #48549, #41902, #62188, #16640, #63808, #9254, #9573, #19593, #49532, #49215, #3329, #29537, #8953, #44843, #3970, #29236, #3000, #34207, #24234 ),
 .UNSPECIFIED., .F., .F.,
 ( 4, 2, 2, 2, 2, 2, 2, 2, 2, 2, 2, 2, 4 ),
 ( 0.02207550202482942009, 0.02483637361899842730, 0.02621680941608292917, 0.02759724521316743451, 0.03035811680733644519, 0.03173855260442095400, 0.03311898840150546280, 0.03587985999567448736, 0.03864073158984350498, 0.04002116738692802073, 0.04140160318401252953, 0.04278203898109704528, 0.04416247477818155409 ),
 .UNSPECIFIED. ) ;
#37680=CARTESIAN_POINT ( 'NONE',  ( 25.00000000000000355, -9.999999999999998224, 5.000000000000000888 ) ) ;
#37687=CARTESIAN_POINT ( 'NONE',  ( -5.261125060311115931, -26.02247534669140094, 15.21511059005040423 ) ) ;
#37771=CARTESIAN_POINT ( 'NONE',  ( -19.56743653832047158, -30.00000000000000355, 5.000000000000000888 ) ) ;
#37773=CARTESIAN_POINT ( 'NONE',  ( -35.62304844322794395, -2.500997609376294228, -21.53526926371173289 ) ) ;
#37781=VERTEX_POINT ( 'NONE', #10743 ) ;
#37868=DIRECTION ( 'NONE',  ( 0.000000000000000000, 0.000000000000000000, -1.000000000000000000 ) ) ;
#37871=AXIS2_PLACEMENT_3D ( 'NONE', #43059, #63338, #13141 ) ;
#37900=CARTESIAN_POINT ( 'NONE',  ( 25.00000000000000711, -3.797884998337192286, -24.00000000000000000 ) ) ;
#37984=CARTESIAN_POINT ( 'NONE',  ( 0.000000000000000000, -30.50000000000000000, -14.13397459621556251 ) ) ;
#37992=VERTEX_POINT ( 'NONE', #29628 ) ;
#37996=DIRECTION ( 'NONE',  ( 0.2475719085175094591, 0.000000000000000000, -0.9688695217174487784 ) ) ;
#37999=CARTESIAN_POINT ( 'NONE',  ( 16.03117610287102579, -28.25087052915268870, 10.32844618003480619 ) ) ;
#38014=ORIENTED_EDGE ( 'NONE', *, *, #10978, .F. ) ;
#38062=AXIS2_PLACEMENT_3D ( 'NONE', #53083, #8505, #3214 ) ;
#38084=CARTESIAN_POINT ( 'NONE',  ( 3.168054457075969665, -30.71813892570239801, 15.09231838820068106 ) ) ;
#38086=CARTESIAN_POINT ( 'NONE',  ( -25.00000000000000355, -3.797884998337192286, -23.99999999999999289 ) ) ;
#38135=CARTESIAN_POINT ( 'NONE',  ( -12.50548042261300097, -29.27747730776674118, -5.013933227252968194 ) ) ;
#38142=EDGE_CURVE ( 'NONE', #39511, #18880, #37388, .T. ) ;
#38200=AXIS2_PLACEMENT_3D ( 'NONE', #10082, #55960, #5101 ) ;
#38218=CARTESIAN_POINT ( 'NONE',  ( -5.894163417175557029, -31.16155000483562176, 14.52685451768251923 ) ) ;
#38219=AXIS2_PLACEMENT_3D ( 'NONE', #34878, #55185, #9617 ) ;
#38225=CARTESIAN_POINT ( 'NONE',  ( 34.90603985575356205, -2.603248520265782684, 21.87429913450488428 ) ) ;
#38231=DIRECTION ( 'NONE',  ( -1.000000000000000000, 0.000000000000000000, 0.000000000000000000 ) ) ;
#38253=CARTESIAN_POINT ( 'NONE',  ( 14.06742311316907212, -34.40796758970419233, -8.422011900746815272 ) ) ;
#38288=AXIS2_PLACEMENT_3D ( 'NONE', #39528, #59827, #60142 ) ;
#38296=DIRECTION ( 'NONE',  ( 0.000000000000000000, 0.000000000000000000, 1.000000000000000000 ) ) ;
#38326=CARTESIAN_POINT ( 'NONE',  ( 18.66975156949834513, -28.88996333714986875, 7.079161351701957372 ) ) ;
#38338=CARTESIAN_POINT ( 'NONE',  ( 15.69195845145067736, -33.00000000000000000, 4.009712365929969380 ) ) ;
#38363=VERTEX_POINT ( 'NONE', #27759 ) ;
#38364=EDGE_CURVE ( 'NONE', #4569, #14095, #19370, .T. ) ;
#38408=CARTESIAN_POINT ( 'NONE',  ( -37.25000000000000711, -27.21021009056489603, 4.499999999999997335 ) ) ;
#38419=ORIENTED_EDGE ( 'NONE', *, *, #7894, .T. ) ;
#38422=CARTESIAN_POINT ( 'NONE',  ( -13.91099446267133999, -33.59051099066034851, 9.908177736482725706 ) ) ;
#38426=CARTESIAN_POINT ( 'NONE',  ( -28.15855999187489189, -3.461419147680624864, -23.80441447217193485 ) ) ;
#38475=CARTESIAN_POINT ( 'NONE',  ( -1.046707184715866212, -25.73493584727765082, -15.64955084339668012 ) ) ;
#38506=CARTESIAN_POINT ( 'NONE',  ( 0.000000000000000000, -30.00000000000000000, -15.00000000000000000 ) ) ;
#38509=AXIS2_PLACEMENT_3D ( 'NONE', #11840, #6549, #5917 ) ;
#38522=DIRECTION ( 'NONE',  ( -0.000000000000000000, 1.000000000000000000, -0.000000000000000000 ) ) ;
#38545=CARTESIAN_POINT ( 'NONE',  ( -16.02919692786944239, -28.24921752684737086, -10.30002093107130356 ) ) ;
#38549=CARTESIAN_POINT ( 'NONE',  ( 0.000000000000000000, -45.00000000000000000, 0.000000000000000000 ) ) ;
#38558=DIRECTION ( 'NONE',  ( 0.000000000000000000, 0.000000000000000000, 1.000000000000000000 ) ) ;
#38572=CARTESIAN_POINT ( 'NONE',  ( -25.00000000000000355, -30.00000000000000000, 24.00000000000000000 ) ) ;
#38580=ORIENTED_EDGE ( 'NONE', *, *, #45484, .T. ) ;
#38604=CARTESIAN_POINT ( 'NONE',  ( -15.60798173055017912, -34.17470894020297578, -7.727686298000182141 ) ) ;
#38627=DIRECTION ( 'NONE',  ( 0.000000000000000000, 1.000000000000000000, 0.000000000000000000 ) ) ;
#38631=VECTOR ( 'NONE', #53014, 1000.000000000000000 ) ;
#38654=CARTESIAN_POINT ( 'NONE',  ( 22.00000000000000711, -20.00000000000000000, -1.499999999999998002 ) ) ;
#38675=CARTESIAN_POINT ( 'NONE',  ( 18.18435566811206527, -28.78814669831782780, 7.856426167042674713 ) ) ;
#38736=VERTEX_POINT ( 'NONE', #38654 ) ;
#38752=VERTEX_POINT ( 'NONE', #28343 ) ;
#38758=CARTESIAN_POINT ( 'NONE',  ( -15.30016555129190792, -29.00876116002328686, 11.22753712088974964 ) ) ;
#38773=MECHANICAL_DESIGN_GEOMETRIC_PRESENTATION_REPRESENTATION('',(#48331),#56878);
#38809=CARTESIAN_POINT ( 'NONE',  ( -8.761386526127953545, -26.55543068763903491, -14.32493309394703829 ) ) ;
#38835=SHAPE_REPRESENTATION_RELATIONSHIP ( 'NONE' , 'NONE' ,  #29683, #4012 ) ;
#38851=DIRECTION ( 'NONE',  ( 0.000000000000000000, 0.000000000000000000, -1.000000000000000000 ) ) ;
#38859=LINE ( 'NONE', #63774, #60336 ) ;
#38916=AXIS2_PLACEMENT_3D ( 'NONE', #15427, #35693, #25089 ) ;
#38935=CARTESIAN_POINT ( 'NONE',  ( -14.24371601685413502, -33.70914924250542555, -9.547107017903027071 ) ) ;
#38939=VERTEX_POINT ( 'NONE', #15648 ) ;
#39061=CARTESIAN_POINT ( 'NONE',  ( 25.00000000000000355, -9.999999999999998224, -5.000000000000000888 ) ) ;
#39067=CARTESIAN_POINT ( 'NONE',  ( -13.26547918569768569, -33.36007533429819460, 10.54465099870296996 ) ) ;
#39080=ORIENTED_EDGE ( 'NONE', *, *, #26896, .T. ) ;
#39086=LINE ( 'NONE', #44393, #61768 ) ;
#39107=ORIENTED_EDGE ( 'NONE', *, *, #63883, .F. ) ;
#39118=CARTESIAN_POINT ( 'NONE',  ( 25.00000000000000355, -30.00000000000000000, 5.000000000000000888 ) ) ;
#39119=CARTESIAN_POINT ( 'NONE',  ( -5.901743774574147672, -31.73659747722650692, -13.63115424678022158 ) ) ;
#39154=DIRECTION ( 'NONE',  ( 0.000000000000000000, -1.000000000000000000, 0.000000000000000000 ) ) ;
#39171=CIRCLE ( 'NONE', #45532, 3.999999999999999112 ) ;
#39172=PRODUCT_DEFINITION_SHAPE ( 'NONE', 'NONE',  #31126 ) ;
#39176=DIRECTION ( 'NONE',  ( 0.000000000000000000, 0.000000000000000000, -1.000000000000000000 ) ) ;
#39235=DIRECTION ( 'NONE',  ( 0.000000000000000000, 0.000000000000000000, -1.000000000000000000 ) ) ;
#39247=B_SPLINE_CURVE_WITH_KNOTS ( 'NONE', 3,
 ( #26976, #47273, #25998, #36278, #41599, #61888, #16347, #36618 ),
 .UNSPECIFIED., .F., .F.,
 ( 4, 2, 2, 4 ),
 ( 0.01093700429183111500, 0.01319343274642247738, 0.01544986120101383975, 0.01996271811019656450 ),
 .UNSPECIFIED. ) ;
#39250=CARTESIAN_POINT ( 'NONE',  ( 41.00000000000000711, -25.03188948156373783, 4.499999999999997335 ) ) ;
#39261=AXIS2_PLACEMENT_3D ( 'NONE', #52406, #43629, #48978 ) ;
#39264=PLANE ( 'NONE',  #48153 ) ;
#39278=CARTESIAN_POINT ( 'NONE',  ( -1.009501604528854735, -26.56249173023641319, -16.21092882686939163 ) ) ;
#39288=ORIENTED_EDGE ( 'NONE', *, *, #54622, .T. ) ;
#39297=CIRCLE ( 'NONE', #35062, 1.500000000000000222 ) ;
#39353=CARTESIAN_POINT ( 'NONE',  ( 33.80171706282990840, -2.756546641835186495, -23.41361577495085200 ) ) ;
#39396=CARTESIAN_POINT ( 'NONE',  ( 1.819964709949660975, -30.58339181399214723, 15.25524951094025639 ) ) ;
#39421=B_SPLINE_CURVE_WITH_KNOTS ( 'NONE', 3,
 ( #55222, #44571, #19976, #9323, #35256, #30593, #55564, #64854, #49918, #10005, #30286, #50900, #19336, #5024, #18, #60876, #15316, #25621, #35592, #24643, #55886, #35900, #4370, #40920, #9022, #44920, #19669, #29304, #46249, #10991, #51889, #10636, #36586, #16310, #20948, #37219, #51575, #41226, #47548, #26599, #56889, #22260, #11314, #11957, #41556, #30928, #61510, #62181 ),
 .UNSPECIFIED., .F., .F.,
 ( 4, 2, 2, 2, 2, 2, 2, 2, 2, 2, 2, 2, 2, 2, 2, 2, 2, 2, 2, 2, 2, 2, 2, 4 ),
 ( 8.673617379884035472E-19, 0.003028155528123375149, 0.004542233292185064893, 0.006056311056246753768, 0.007570388820308435705, 0.009084466584370117642, 0.01211262211249347978, 0.01514077764061684192, 0.01816893316874019712, 0.02119708869686355926, 0.02271116646092524380, 0.02422524422498692487, 0.02725339975311028701, 0.02876747751717196808, 0.03028155528123365262, 0.03330971080935701129, 0.03482378857341869582, 0.03633786633748037342, 0.03936602186560374944, 0.04239417739372711852, 0.04390825515778881000, 0.04542233292185050147, 0.04693641068591217907, 0.04845048844997387055 ),
 .UNSPECIFIED. ) ;
#39445=CARTESIAN_POINT ( 'NONE',  ( 1.074417311476293158, -25.72614907888524982, -15.66246854766675156 ) ) ;
#39478=ORIENTED_EDGE ( 'NONE', *, *, #57273, .F. ) ;
#39511=VERTEX_POINT ( 'NONE', #18573 ) ;
#39528=CARTESIAN_POINT ( 'NONE',  ( 0.000000000000000000, -34.50000000000000000, 0.000000000000000000 ) ) ;
#39579=CARTESIAN_POINT ( 'NONE',  ( -16.81801275797669604, -34.49999999999998579, -5.265606433705287692 ) ) ;
#39610=VECTOR ( 'NONE', #60368, 1000.000000000000000 ) ;
#39646=CARTESIAN_POINT ( 'NONE',  ( -11.31614860309490922, -29.68432482266972272, -9.654990830001235480 ) ) ;
#39654=FACE_OUTER_BOUND ( 'NONE', #36495, .T. ) ;
#39692=CARTESIAN_POINT ( 'NONE',  ( 41.46388549984528282, -1.589384660823696782, -18.83126657550987915 ) ) ;
#39724=CARTESIAN_POINT ( 'NONE',  ( -16.02805653289875920, -28.24868299250882941, 10.29995797863329621 ) ) ;
#39735=CARTESIAN_POINT ( 'NONE',  ( 16.25880638382997745, -34.36679772354796114, 6.546306705357587852 ) ) ;
#39762=CARTESIAN_POINT ( 'NONE',  ( -41.00000000000000711, -1.694065894508600678E-18, 0.000000000000000000 ) ) ;
#39780=ORIENTED_EDGE ( 'NONE', *, *, #63940, .F. ) ;
#39783=CARTESIAN_POINT ( 'NONE',  ( -8.110750208426855679, -28.65453171996802695, -10.34333599818553928 ) ) ;
#39849=EDGE_CURVE ( 'NONE', #33165, #4569, #48036, .T. ) ;
#39895=EDGE_LOOP ( 'NONE', ( #65065, #24114, #28592, #49090 ) ) ;
#39936=DIRECTION ( 'NONE',  ( 0.000000000000000000, 1.000000000000000000, 0.000000000000000000 ) ) ;
#39949=CIRCLE ( 'NONE', #42075, 1.500000000000000222 ) ;
#39961=ORIENTED_EDGE ( 'NONE', *, *, #631, .F. ) ;
#39967=CARTESIAN_POINT ( 'NONE',  ( -0.4406170177989157666, -30.53628804997674706, -15.30998899416534975 ) ) ;
#40011=CARTESIAN_POINT ( 'NONE',  ( -46.64267184946612588, -0.6617291737840982346, -12.54075111122643271 ) ) ;
#40014=CARTESIAN_POINT ( 'NONE',  ( 8.843349564596783452, -31.89871022336353334, 13.45657735392122589 ) ) ;
#40038=CARTESIAN_POINT ( 'NONE',  ( -10.20982488791560883, -26.83227745022078992, 13.82162602233992565 ) ) ;
#40048=CARTESIAN_POINT ( 'NONE',  ( 15.82775651593409627, -34.24354600359715306, 7.361827980272476424 ) ) ;
#40065=CARTESIAN_POINT ( 'NONE',  ( -19.56743653832047158, -33.00000000000000000, 5.000000000000000888 ) ) ;
#40066=DIRECTION ( 'NONE',  ( -1.000000000000000000, -0.000000000000000000, -0.000000000000000000 ) ) ;
#40088=CARTESIAN_POINT ( 'NONE',  ( -11.32744364968826112, -33.39367328239853094, -11.05351320890539668 ) ) ;
#40093=CARTESIAN_POINT ( 'NONE',  ( 17.02556425888772296, -28.50707051634331890, -9.313930266526256219 ) ) ;
#40119=DIRECTION ( 'NONE',  ( 0.000000000000000000, -1.000000000000000000, 0.000000000000000000 ) ) ;
#40205=ADVANCED_FACE ( 'NONE', ( #59859 ), #14285, .T. ) ;
#40243=SURFACE_STYLE_USAGE ( .BOTH. , #19975 ) ;
#40252=VECTOR ( 'NONE', #6473, 1000.000000000000000 ) ;
#40255=CARTESIAN_POINT ( 'NONE',  ( -9.857630741398546448, -27.64257788600498600, -14.42778837489968424 ) ) ;
#40283=CARTESIAN_POINT ( 'NONE',  ( 3.616736114193129126, -30.77385512440640980, -15.02426791487768831 ) ) ;
#40286=ORIENTED_EDGE ( 'NONE', *, *, #36821, .F. ) ;
#40313=AXIS2_PLACEMENT_3D ( 'NONE', #27223, #3280, #2956 ) ;
#40328=CARTESIAN_POINT ( 'NONE',  ( 31.50196089333760696, -3.063567359192289619, 24.19471064305899688 ) ) ;
#40332=CARTESIAN_POINT ( 'NONE',  ( 9.648902782409225054, -32.13880772996252233, 13.06387094875849897 ) ) ;
#40350=VERTEX_POINT ( 'NONE', #4671 ) ;
#40358=CARTESIAN_POINT ( 'NONE',  ( -16.21117406328131594, -35.00000000000000000, 4.142385751841761277 ) ) ;
#40369=CARTESIAN_POINT ( 'NONE',  ( 9.992127424269058977, -32.24574823824644909, 12.88148438038762400 ) ) ;
#40394=AXIS2_PLACEMENT_3D ( 'NONE', #6898, #36134, #41803 ) ;
#40423=CARTESIAN_POINT ( 'NONE',  ( 9.461050110694847248, -32.74574823825055603, -12.19700847635464669 ) ) ;
#40492=ORIENTED_EDGE ( 'NONE', *, *, #49447, .T. ) ;
#40535=CIRCLE ( 'NONE', #62842, 4.500000000000000888 ) ;
#40559=CARTESIAN_POINT ( 'NONE',  ( 0.9972908435452138010, -25.72582856205513480, 15.66294124711422775 ) ) ;
#40561=FACE_OUTER_BOUND ( 'NONE', #10491, .T. ) ;
#40572=DIRECTION ( 'NONE',  ( -1.000000000000000000, 0.000000000000000000, 0.000000000000000000 ) ) ;
#40604=AXIS2_PLACEMENT_3D ( 'NONE', #62169, #6321, #21269 ) ;
#40607=CARTESIAN_POINT ( 'NONE',  ( 46.85239813472878723, -0.6216812786252600143, -9.954194587011503614 ) ) ;
#40625=CARTESIAN_POINT ( 'NONE',  ( -6.778443870680789907, -27.08263571440718209, -15.40204062588007083 ) ) ;
#40670=CARTESIAN_POINT ( 'NONE',  ( 49.43099673984273323, -0.1154732602011161596, -5.319553669056248602 ) ) ;
#40675=EDGE_CURVE ( 'NONE', #64767, #15355, #5906, .T. ) ;
#40678=CARTESIAN_POINT ( 'NONE',  ( 13.92922077006917014, -33.59874296436205299, 9.921733781850763378 ) ) ;
#40682=EDGE_CURVE ( 'NONE', #33165, #17827, #45131, .T. ) ;
#40705=CARTESIAN_POINT ( 'NONE',  ( -7.119438362040798829, -32.04078451673858297, 13.23628618373588317 ) ) ;
#40717=CARTESIAN_POINT ( 'NONE',  ( 7.310206959902322055, -27.15910349781274391, 15.27822828334930350 ) ) ;
#40737=EDGE_CURVE ( 'NONE', #54875, #32724, #7786, .T. ) ;
#40739=EDGE_LOOP ( 'NONE', ( #27267, #55744, #57424, #15615, #53460, #19578 ) ) ;
#40743=DIRECTION ( 'NONE',  ( 0.000000000000000000, 1.000000000000000000, -0.000000000000000000 ) ) ;
#40759=AXIS2_PLACEMENT_3D ( 'NONE', #18869, #24170, #34776 ) ;
#40773=CARTESIAN_POINT ( 'NONE',  ( 12.50310467286144167, -29.27802453453052323, -5.021082754746766241 ) ) ;
#40804=ORIENTED_EDGE ( 'NONE', *, *, #631, .T. ) ;
#40884=EDGE_LOOP ( 'NONE', ( #20081, #63215, #19734, #48322, #50643, #1145 ) ) ;
#40892=EDGE_LOOP ( 'NONE', ( #20750, #2723, #37245, #4363 ) ) ;
#40919=CARTESIAN_POINT ( 'NONE',  ( 19.22959543997423637, -28.98134239863147954, -5.957279114860658531 ) ) ;
#40920=CARTESIAN_POINT ( 'NONE',  ( 1.014403380171174041, -26.55354399125274867, 16.22408933255776731 ) ) ;
#40956=CARTESIAN_POINT ( 'NONE',  ( 7.085269882676524134, -28.78331678329937304, -12.46778293907698121 ) ) ;
#40959=DIRECTION ( 'NONE',  ( -0.000000000000000000, -0.000000000000000000, -1.000000000000000000 ) ) ;
#40969=DIRECTION ( 'NONE',  ( 0.000000000000000000, -0.000000000000000000, 1.000000000000000000 ) ) ;
#40970=DIRECTION ( 'NONE',  ( 0.000000000000000000, 1.000000000000000000, 0.000000000000000000 ) ) ;
#41025=CARTESIAN_POINT ( 'NONE',  ( -5.876491384319547429, -28.27454061773107696, 11.46433771796954382 ) ) ;
#41030=ORIENTED_EDGE ( 'NONE', *, *, #48792, .F. ) ;
#41036=CARTESIAN_POINT ( 'NONE',  ( 12.91449914267798960, -28.36597991684631026, 12.93464570467208752 ) ) ;
#41061=LINE ( 'NONE', #65661, #9557 ) ;
#41075=CARTESIAN_POINT ( 'NONE',  ( -8.419536088387953754, -32.40770164631213390, -12.72556558505306157 ) ) ;
#41080=CARTESIAN_POINT ( 'NONE',  ( 19.27363075669222425, -28.98570064806743929, -5.846556568011616939 ) ) ;
#41141=CARTESIAN_POINT ( 'NONE',  ( 41.00000000000000711, -1.694065894508600678E-18, 0.000000000000000000 ) ) ;
#41186=CARTESIAN_POINT ( 'NONE',  ( -15.59741926310024773, -34.17135967094577609, 7.744809993482618005 ) ) ;
#41191=CARTESIAN_POINT ( 'NONE',  ( -26.58307969160926021, -3.634951060761377750, -23.96081192854774500 ) ) ;
#41203=CARTESIAN_POINT ( 'NONE',  ( -3.987543989681922696, -25.89241204356462589, 15.41372194231675330 ) ) ;
#41213=CONICAL_SURFACE ( 'NONE', #28452, 15.00000000000000000, 0.5235987755983000369 ) ;
#41225=CARTESIAN_POINT ( 'NONE',  ( -9.737135312703241397, -26.73636926326595642, -14.00099174170044058 ) ) ;
#41226=CARTESIAN_POINT ( 'NONE',  ( 14.99320290036091308, -28.92253633446381400, 11.50449902612425923 ) ) ;
#41242=AXIS2_PLACEMENT_3D ( 'NONE', #18258, #28540, #33543 ) ;
#41250=CARTESIAN_POINT ( 'NONE',  ( 49.00067463083239971, -0.2018647702349731232, 0.7653472444253841545 ) ) ;
#41266=CARTESIAN_POINT ( 'NONE',  ( 13.85759530760289060, -30.12605952702162426, -5.992721990255803988 ) ) ;
#41274=CARTESIAN_POINT ( 'NONE',  ( 37.25000000000000711, -45.00200000000000244, 4.499999999999997335 ) ) ;
#41345=CARTESIAN_POINT ( 'NONE',  ( -4.228765754682470401, -25.91303510919334485, 15.38236557491807766 ) ) ;
#41356=CARTESIAN_POINT ( 'NONE',  ( 17.05023968204111284, -34.49999999999999289, 4.356789313881303194 ) ) ;
#41367=VERTEX_POINT ( 'NONE', #55935 ) ;
#41370=CARTESIAN_POINT ( 'NONE',  ( -25.00000000000000355, -28.99999999999999645, 1.530808498934191521E-15 ) ) ;
#41392=CARTESIAN_POINT ( 'NONE',  ( 9.537768711910022290, -32.77116127932499268, 12.15562491790719513 ) ) ;
#41393=CIRCLE ( 'NONE', #40313, 1.500000000000000444 ) ;
#41398=CARTESIAN_POINT ( 'NONE',  ( -25.00000000000000355, -9.999999999999998224, -24.00000000000000000 ) ) ;
#41400=CARTESIAN_POINT ( 'NONE',  ( 13.20768530587737288, -34.09315906254132500, -9.434917751661075158 ) ) ;
#41446=DIRECTION ( 'NONE',  ( 1.000000000000000000, 0.000000000000000000, -0.000000000000000000 ) ) ;
#41468=ORIENTED_EDGE ( 'NONE', *, *, #59595, .T. ) ;
#41514=CARTESIAN_POINT ( 'NONE',  ( -19.30028543097103011, -30.00000000000000355, 5.909123879098597598 ) ) ;
#41515=VERTEX_POINT ( 'NONE', #17596 ) ;
#41517=CARTESIAN_POINT ( 'NONE',  ( -17.92531974009792606, -29.71422580122515456, -8.391737566681648275 ) ) ;
#41555=CARTESIAN_POINT ( 'NONE',  ( 3.474069148988125466, -25.85800187936593986, -15.46552914816620827 ) ) ;
#41556=CARTESIAN_POINT ( 'NONE',  ( 18.81741048081455503, -29.91393404465042849, 6.911695701493934862 ) ) ;
#41568=VECTOR ( 'NONE', #57359, 1000.000000000000000 ) ;
#41584=CARTESIAN_POINT ( 'NONE',  ( 40.83349710434615076, -1.696348104764147768, 18.10529304745326584 ) ) ;
#41586=ADVANCED_FACE ( 'NONE', ( #49497 ), #3285, .T. ) ;
#41599=CARTESIAN_POINT ( 'NONE',  ( 37.25000000000000711, -27.56270118634207122, 0.7455576661145019157 ) ) ;
#41605=CARTESIAN_POINT ( 'NONE',  ( 12.84304429912246981, -30.00680404000052448, -7.859709520792301340 ) ) ;
#41613=CARTESIAN_POINT ( 'NONE',  ( -9.179144435730854923, -32.64956785249903959, 12.36195000407851907 ) ) ;
#41653=DIRECTION ( 'NONE',  ( 0.000000000000000000, 0.000000000000000000, -1.000000000000000000 ) ) ;
#41686=CARTESIAN_POINT ( 'NONE',  ( -1.046707184715866212, -25.73493584727765082, 15.64955084339668012 ) ) ;
#41711=CARTESIAN_POINT ( 'NONE',  ( -25.00000000000000355, -30.00000000000000000, 5.000000000000000888 ) ) ;
#41730=EDGE_CURVE ( 'NONE', #939, #659, #15267, .T. ) ;
#41769=DIRECTION ( 'NONE',  ( 0.000000000000000000, 0.000000000000000000, 1.000000000000000000 ) ) ;
#41803=DIRECTION ( 'NONE',  ( -1.000000000000000000, 0.000000000000000000, 0.000000000000000000 ) ) ;
#41804=ORIENTED_EDGE ( 'NONE', *, *, #1827, .F. ) ;
#41823=B_SPLINE_CURVE_WITH_KNOTS ( 'NONE', 3,
 ( #39250, #49583, #64514, #63861 ),
 .UNSPECIFIED., .F., .F.,
 ( 4, 4 ),
 ( 0.007620068080905808769, 0.01192914805994312565 ),
 .UNSPECIFIED. ) ;
#41873=PLANE ( 'NONE',  #2344 ) ;
#41898=CIRCLE ( 'NONE', #64248, 19.00000000000000000 ) ;
#41902=CARTESIAN_POINT ( 'NONE',  ( 7.188828048469327214, -31.44854185097339894, -14.13838964164549417 ) ) ;
#41910=CIRCLE ( 'NONE', #62098, 1.500000000000000444 ) ;
#41914=CARTESIAN_POINT ( 'NONE',  ( 41.38732981120778476, -1.602042930228849249, -17.55180477253563964 ) ) ;
#41930=CARTESIAN_POINT ( 'NONE',  ( 13.40144019692491995, -30.08877117594819595, -6.927253557473251888 ) ) ;
#41938=CARTESIAN_POINT ( 'NONE',  ( -3.498383876424262517, -31.27426290440205747, 14.18200193795962605 ) ) ;
#41940=DIRECTION ( 'NONE',  ( -0.2475719085175105416, 8.403603522408387294E-16, -0.9688695217174485563 ) ) ;
#41947=VECTOR ( 'NONE', #26604, 1000.000000000000000 ) ;
#42005=CARTESIAN_POINT ( 'NONE',  ( 3.448218607682480563, -27.97504209443001955, 12.21548802405080991 ) ) ;
#42054=CARTESIAN_POINT ( 'NONE',  ( -25.00000000000000355, -30.00000000000000000, -5.000000000000000888 ) ) ;
#42060=DIRECTION ( 'NONE',  ( -1.000000000000000000, -0.000000000000000000, 0.000000000000000000 ) ) ;
#42065=ORIENTED_EDGE ( 'NONE', *, *, #27794, .T. ) ;
#42075=AXIS2_PLACEMENT_3D ( 'NONE', #18032, #43610, #38296 ) ;
#42161=CIRCLE ( 'NONE', #31590, 20.00000000000000000 ) ;
#42173=ORIENTED_EDGE ( 'NONE', *, *, #63883, .T. ) ;
#42200=DIRECTION ( 'NONE',  ( 0.000000000000000000, 0.000000000000000000, 1.000000000000000000 ) ) ;
#42235=CARTESIAN_POINT ( 'NONE',  ( 15.30590914263659386, -29.00884126188377365, -11.24874127360776654 ) ) ;
#42236=CARTESIAN_POINT ( 'NONE',  ( -37.25000000000000711, -1.853910857666116187E-16, -1.500000000000000222 ) ) ;
#42239=CARTESIAN_POINT ( 'NONE',  ( 17.05023968204110574, -34.50000000000000000, -4.356789313881336057 ) ) ;
#42240=EDGE_LOOP ( 'NONE', ( #20777, #53211, #7587, #56370 ) ) ;
#42252=EDGE_CURVE ( 'NONE', #31959, #65704, #9559, .T. ) ;
#42313=CARTESIAN_POINT ( 'NONE',  ( 7.919433923537877895, -32.26502814485947823, 12.92562328492908286 ) ) ;
#42421=ORIENTED_EDGE ( 'NONE', *, *, #14981, .F. ) ;
#42432=ORIENTED_EDGE ( 'NONE', *, *, #45930, .T. ) ;
#42451=CARTESIAN_POINT ( 'NONE',  ( -16.37486794060187734, -28.33944867960597236, -9.978426449060183501 ) ) ;
#42479=( LENGTH_UNIT ( ) NAMED_UNIT ( * ) SI_UNIT ( .MILLI., .METRE. ) );
#42488=CARTESIAN_POINT ( 'NONE',  ( -13.40508024069041326, -30.08919203117021368, -6.920461462856672519 ) ) ;
#42499=CARTESIAN_POINT ( 'NONE',  ( -1.318817192132426526E-11, -30.53649492335491544, -15.30974548841782834 ) ) ;
#42577=CARTESIAN_POINT ( 'NONE',  ( 19.56743653832047158, -33.00000000000000000, -5.000000000000017764 ) ) ;
#42605=AXIS2_PLACEMENT_3D ( 'NONE', #6800, #1810, #8106 ) ;
#42609=CARTESIAN_POINT ( 'NONE',  ( 11.20797324838622444, -27.95044230146133302, -13.82289656124156885 ) ) ;
#42643=CARTESIAN_POINT ( 'NONE',  ( -0.4156926711315701573, -31.03628804997841684, 14.44394305974772408 ) ) ;
#42656=AXIS2_PLACEMENT_3D ( 'NONE', #15566, #62119, #16572 ) ;
#42676=DIRECTION ( 'NONE',  ( 0.000000000000000000, 0.000000000000000000, -1.000000000000000000 ) ) ;
#42691=( BOUNDED_SURFACE ( )  B_SPLINE_SURFACE ( 3, 2, ( 
 ( #62452, #12252, #7254 ),
 ( #11280, #37184, #11595 ),
 ( #6299, #6951, #52184 ),
 ( #31549, #6631, #11920 ),
 ( #36550, #58146, #41517 ),
 ( #62786, #32197, #22228 ),
 ( #2295, #42488, #17254 ),
 ( #37528, #22572, #42834 ),
 ( #57833, #61810, #63125 ),
 ( #12561, #32842, #5990 ),
 ( #26246, #46520, #34639 ),
 ( #24686, #39646, #14673 ),
 ( #24345, #25663, #20681 ),
 ( #15011, #29650, #29990 ),
 ( #45957, #9060, #9701 ),
 ( #60576, #14037, #54642 ),
 ( #29340, #64900, #49637 ),
 ( #45606, #4077, #65244 ),
 ( #55924, #412, #40625 ),
 ( #34956, #20341, #50302 ),
 ( #35630, #55262, #35297 ),
 ( #59946, #44963, #65547 ),
 ( #10355, #19712, #4755 ),
 ( #5391, #44610, #50943 ),
 ( #39967, #60249, #25017 ),
 ( #45289, #59608, #57 ),
 ( #34328, #19379, #20017 ),
 ( #55610, #14367, #54935 ),
 ( #40283, #10046, #9365 ),
 ( #30327, #49956, #50620 ),
 ( #4416, #60920, #5066 ),
 ( #25329, #15357, #30632 ),
 ( #5735, #40956, #52596 ),
 ( #61892, #7021, #47585 ),
 ( #2031, #46598, #26002 ),
 ( #1054, #21323, #35938 ),
 ( #1718, #21983, #26982 ),
 ( #20985, #36623, #36283 ),
 ( #27291, #56240, #15662 ),
 ( #46286, #61549, #42235 ),
 ( #51612, #41605, #6058 ),
 ( #26316, #41930, #16351 ),
 ( #61236, #47277, #56929 ),
 ( #15995, #41266, #21676 ),
 ( #11348, #10682, #62528 ),
 ( #56589, #31618, #727 ),
 ( #30969, #51285, #51931 ),
 ( #11031, #6373, #31310 ),
 ( #26641, #46934, #1395 ),
 ( #62215, #16666, #36939 ) ),
 .UNSPECIFIED., .F., .F., .F. ) 
 B_SPLINE_SURFACE_WITH_KNOTS ( ( 4, 2, 2, 2, 2, 2, 2, 2, 2, 2, 2, 2, 2, 2, 2, 2, 2, 2, 2, 2, 2, 2, 2, 2, 4 ),
 ( 3, 3 ),
 ( 0.06047842900482980344, 0.06367705432712368607, 0.06527636698827063433, 0.06687567964941756871, 0.06847499231056451696, 0.07007430497171146522, 0.07327293029400534785, 0.07647155561629923048, 0.07807086827744617874, 0.07967018093859312700, 0.08286880626088700963, 0.08446811892203395788, 0.08606743158318089226, 0.08926605690547478877, 0.09086536956662172315, 0.09246468222776867141, 0.09566330755006255404, 0.09726262021120950230, 0.09886193287235645055, 0.1020605581946503332, 0.1052591835169442158, 0.1068584961780911641, 0.1084578088392381123, 0.1100571215003850467, 0.1116564341615319950 ),
 ( 0.000000000000000000, 1.000000000000000000 ),
 .UNSPECIFIED. ) 
 GEOMETRIC_REPRESENTATION_ITEM ( )  RATIONAL_B_SPLINE_SURFACE ( (
 ( 1.000000000000000000, 0.4999999999999997224, 1.000000000000000000),
 ( 1.000000000000000000, 0.5048840838053595403, 1.000000000000000000),
 ( 1.000000000000000000, 0.5132072642500214998, 1.000000000000000000),
 ( 1.000000000000000000, 0.5290214861663712353, 1.000000000000000000),
 ( 1.000000000000000000, 0.5348648783786204008, 1.000000000000000000),
 ( 1.000000000000000000, 0.5473516051742154387, 1.000000000000000000),
 ( 1.000000000000000000, 0.5539126387907835625, 1.000000000000000000),
 ( 1.000000000000000000, 0.5674101295480111773, 1.000000000000000000),
 ( 1.000000000000000000, 0.5743474342085095330, 1.000000000000000000),
 ( 1.000000000000000000, 0.5883951384280732277, 1.000000000000000000),
 ( 1.000000000000000000, 0.5955302209472060904, 1.000000000000000000),
 ( 1.000000000000000000, 0.6167715304226100148, 1.000000000000000000),
 ( 1.000000000000000000, 0.6305661306844096980, 1.000000000000000000),
 ( 1.000000000000000000, 0.6565125894475725143, 1.000000000000000000),
 ( 1.000000000000000000, 0.6686743926052454157, 1.000000000000000000),
 ( 1.000000000000000000, 0.6851014456086110815, 1.000000000000000000),
 ( 1.000000000000000000, 0.6902475665163220198, 1.000000000000000000),
 ( 1.000000000000000000, 0.6997062435424069582, 1.000000000000000000),
 ( 1.000000000000000000, 0.7040363771868437537, 1.000000000000000000),
 ( 1.000000000000000000, 0.7157418617800307414, 1.000000000000000000),
 ( 1.000000000000000000, 0.7218341033859928535, 1.000000000000000000),
 ( 1.000000000000000000, 0.7280280015705831165, 1.000000000000000000),
 ( 1.000000000000000000, 0.7296036051600910399, 1.000000000000000000),
 ( 1.000000000000000000, 0.7316818214127936981, 1.000000000000000000),
 ( 1.000000000000000000, 0.7321927565546040295, 1.000000000000000000),
 ( 1.000000000000000000, 0.7321641879719948953, 1.000000000000000000),
 ( 1.000000000000000000, 0.7300624469249552551, 1.000000000000000000),
 ( 1.000000000000000000, 0.7238943330025175982, 1.000000000000000000),
 ( 1.000000000000000000, 0.7213359435419578469, 1.000000000000000000),
 ( 1.000000000000000000, 0.7152343487864250005, 1.000000000000000000),
 ( 1.000000000000000000, 0.7117056589944237288, 1.000000000000000000),
 ( 1.000000000000000000, 0.6999072021060018800, 1.000000000000000000),
 ( 1.000000000000000000, 0.6903911339385546686, 1.000000000000000000),
 ( 1.000000000000000000, 0.6741089150888935899, 1.000000000000000000),
 ( 1.000000000000000000, 0.6683461163769471858, 1.000000000000000000),
 ( 1.000000000000000000, 0.6562237482356158003, 1.000000000000000000),
 ( 1.000000000000000000, 0.6498375142660285375, 1.000000000000000000),
 ( 1.000000000000000000, 0.6302143011363016134, 1.000000000000000000),
 ( 1.000000000000000000, 0.6164540672887561801, 1.000000000000000000),
 ( 1.000000000000000000, 0.5885848209491306715, 1.000000000000000000),
 ( 1.000000000000000000, 0.5744580946949985334, 1.000000000000000000),
 ( 1.000000000000000000, 0.5540565490002123950, 1.000000000000000000),
 ( 1.000000000000000000, 0.5474350731751662646, 1.000000000000000000),
 ( 1.000000000000000000, 0.5350293539660013753, 1.000000000000000000),
 ( 1.000000000000000000, 0.5292092555093375061, 1.000000000000000000),
 ( 1.000000000000000000, 0.5186171472262197657, 1.000000000000000000),
 ( 1.000000000000000000, 0.5138445523878424348, 1.000000000000000000),
 ( 1.000000000000000000, 0.5056909436241939781, 1.000000000000000000),
 ( 1.000000000000000000, 0.5023956439952818043, 1.000000000000000000),
 ( 1.000000000000000000, 0.4999999999999995004, 1.000000000000000000) ) ) 
 REPRESENTATION_ITEM ( '' )  SURFACE ( )  );
#42744=CARTESIAN_POINT ( 'NONE',  ( -46.51586683006346590, -0.6857498399870952666, 10.66240463596387578 ) ) ;
#42802=CARTESIAN_POINT ( 'NONE',  ( -15.30016555129190792, -28.05832310202213620, -10.91616026484521385 ) ) ;
#42834=CARTESIAN_POINT ( 'NONE',  ( -16.37486794060188444, -29.30468282063774765, -10.24044889374801315 ) ) ;
#42870=ORIENTED_EDGE ( 'NONE', *, *, #1827, .T. ) ;
#42872=CARTESIAN_POINT ( 'NONE',  ( -16.73721172569806015, -28.43318523521388030, -9.619723400408265235 ) ) ;
#42904=AXIS2_PLACEMENT_3D ( 'NONE', #63619, #2140, #42676 ) ;
#42918=CIRCLE ( 'NONE', #52541, 3.000000000000000444 ) ;
#42929=CARTESIAN_POINT ( 'NONE',  ( 1.744217550858792265, -31.08480052993691345, -14.39239673296543920 ) ) ;
#42950=CYLINDRICAL_SURFACE ( 'NONE', #57691, 19.00000000000000000 ) ;
#42962=CARTESIAN_POINT ( 'NONE',  ( 7.002886717044651377, -27.11012757947470320, -15.35900505431295926 ) ) ;
#42966=DIRECTION ( 'NONE',  ( 0.000000000000000000, -1.000000000000000000, 0.000000000000000000 ) ) ;
#42980=COLOUR_RGB ( '', 0.31764706, 0.68627451, 0.89019608) ;
#43000=ORIENTED_EDGE ( 'NONE', *, *, #41730, .T. ) ;
#43036=VERTEX_POINT ( 'NONE', #25480 ) ;
#43059=CARTESIAN_POINT ( 'NONE',  ( 41.00000000000000711, -45.00200000000000244, 4.499999999999997335 ) ) ;
#43061=DIRECTION ( 'NONE',  ( 0.000000000000000000, 0.000000000000000000, 1.000000000000000000 ) ) ;
#43062=ADVANCED_FACE ( 'NONE', ( #45429, #10186 ), #19222, .F. ) ;
#43078=CARTESIAN_POINT ( 'NONE',  ( -48.61333473403968952, -0.2789806315675443793, -4.308813575818139618 ) ) ;
#43079=FACE_OUTER_BOUND ( 'NONE', #31945, .T. ) ;
#43081=CIRCLE ( 'NONE', #623, 17.19615242270663558 ) ;
#43093=CARTESIAN_POINT ( 'NONE',  ( -37.25000000000001421, -27.53407839942726554, 1.504154570186529760 ) ) ;
#43125=CARTESIAN_POINT ( 'NONE',  ( -11.18139917412363182, -29.23077454460525360, -7.530122743832658117 ) ) ;
#43159=DIRECTION ( 'NONE',  ( -0.9688695217174487784, 0.000000000000000000, 0.2475719085175093481 ) ) ;
#43169=EDGE_CURVE ( 'NONE', #12741, #26603, #26619, .T. ) ;
#43214=EDGE_LOOP ( 'NONE', ( #32615, #56985, #63540, #21625 ) ) ;
#43216=ORIENTED_EDGE ( 'NONE', *, *, #7030, .F. ) ;
#43275=ADVANCED_FACE ( 'NONE', ( #63021 ), #17482, .F. ) ;
#43278=CARTESIAN_POINT ( 'NONE',  ( 1.014403380171158497, -26.55354399125275577, -16.22408933255776731 ) ) ;
#43341=TOROIDAL_SURFACE ( 'NONE', #11487, 5.000000000000000888, 19.00000000000000000 ) ;
#43367=CARTESIAN_POINT ( 'NONE',  ( 25.00000000000000355, -9.999999999999998224, -5.000000000000000888 ) ) ;
#43396=CARTESIAN_POINT ( 'NONE',  ( -2.264138978095803445, -30.62783502483855358, 15.20150737401304575 ) ) ;
#43401=DIRECTION ( 'NONE',  ( 1.000000000000000000, 0.000000000000000000, -0.000000000000000000 ) ) ;
#43402=ORIENTED_EDGE ( 'NONE', *, *, #14446, .F. ) ;
#43448=CARTESIAN_POINT ( 'NONE',  ( -1.729917593620911020, -27.85289612474432275, -12.49635169356267106 ) ) ;
#43471=( NAMED_UNIT ( * ) SI_UNIT ( $, .STERADIAN. ) SOLID_ANGLE_UNIT ( ) );
#43509=CIRCLE ( 'NONE', #48858, 18.99999999999999645 ) ;
#43527=ADVANCED_FACE ( 'NONE', ( #4822 ), #27237, .T. ) ;
#43535=TOROIDAL_SURFACE ( 'NONE', #38219, 20.19615242270663558, 4.000000000000000000 ) ;
#43541=VERTEX_POINT ( 'NONE', #6441 ) ;
#43544=LINE ( 'NONE', #38572, #18378 ) ;
#43572=CARTESIAN_POINT ( 'NONE',  ( -18.83018139755647269, -28.92741097219608903, 6.858339499770058190 ) ) ;
#43588=EDGE_LOOP ( 'NONE', ( #26470, #61584, #5368, #61296 ) ) ;
#43604=CARTESIAN_POINT ( 'NONE',  ( 13.39083528062608330, -28.49171679073736740, -12.64377518253358978 ) ) ;
#43610=DIRECTION ( 'NONE',  ( -1.000000000000000000, 0.000000000000000000, 0.000000000000000000 ) ) ;
#43629=DIRECTION ( 'NONE',  ( -1.000000000000000000, 0.000000000000000000, 0.000000000000000000 ) ) ;
#43690=( BOUNDED_SURFACE ( )  B_SPLINE_SURFACE ( 3, 2, ( 
 ( #37771, #51540, #46517 ),
 ( #41514, #7171, #21239 ),
 ( #15592, #30883, #46211 ),
 ( #47751, #53060, #2201 ),
 ( #653, #58064, #41186 ),
 ( #48094, #63036, #12478 ),
 ( #36194, #32753, #56502 ),
 ( #64341, #58387, #24117 ),
 ( #24428, #49085, #38422 ),
 ( #38758, #48423, #39067 ),
 ( #14123, #44071, #33101 ),
 ( #59057, #7854, #49719 ),
 ( #28769, #19123, #53407 ),
 ( #3536, #59363, #13466 ),
 ( #53732, #23810, #18809 ),
 ( #23460, #59698, #33748 ),
 ( #29423, #2875, #54052 ),
 ( #23131, #3193, #8486 ),
 ( #64993, #43737, #4166 ),
 ( #18505, #13785, #34075 ),
 ( #28128, #64018, #34418 ),
 ( #13159, #54393, #43396 ),
 ( #63672, #8826, #29115 ),
 ( #54718, #18149, #8167 ),
 ( #33441, #58737, #44702 ),
 ( #28438, #48742, #49419 ),
 ( #3859, #44375, #39396 ),
 ( #64654, #9140, #38084 ),
 ( #12813, #46367, #51379 ),
 ( #56330, #4836, #10442 ),
 ( #25420, #45055, #29737 ),
 ( #40717, #35042, #50706 ),
 ( #25102, #5830, #36033 ),
 ( #5493, #15441, #45371 ),
 ( #501, #65631, #46049 ),
 ( #55355, #15108, #30409 ),
 ( #61319, #20107, #40369 ),
 ( #41036, #34721, #60673 ),
 ( #35387, #20766, #9792 ),
 ( #45699, #30722, #10779 ),
 ( #4506, #50390, #56006 ),
 ( #25759, #60335, #55020 ),
 ( #19793, #24776, #9453 ),
 ( #14763, #50046, #55694 ),
 ( #26091, #65326, #40048 ),
 ( #10131, #159, #39735 ),
 ( #5152, #20440, #14444 ),
 ( #61007, #31067, #30077 ),
 ( #35709, #51030, #60027 ),
 ( #15753, #19465, #41356 ) ),
 .UNSPECIFIED., .F., .F., .F. ) 
 B_SPLINE_SURFACE_WITH_KNOTS ( ( 4, 2, 2, 2, 2, 2, 2, 2, 2, 2, 2, 2, 2, 2, 2, 2, 2, 2, 2, 2, 2, 2, 2, 2, 4 ),
 ( 3, 3 ),
 ( 0.06047842900482980344, 0.06367705432712369995, 0.06527636698827063433, 0.06687567964941758258, 0.06847499231056453084, 0.07007430497171146522, 0.07327293029400536173, 0.07647155561629924436, 0.07807086827744619262, 0.07967018093859312700, 0.08286880626088702351, 0.08446811892203395788, 0.08606743158318090614, 0.08926605690547478877, 0.09086536956662173703, 0.09246468222776868529, 0.09566330755006256792, 0.09726262021120951617, 0.09886193287235645055, 0.1020605581946503471, 0.1052591835169442297, 0.1068584961780911780, 0.1084578088392381123, 0.1100571215003850606, 0.1116564341615320088 ),
 ( 0.000000000000000000, 1.000000000000000000 ),
 .UNSPECIFIED. ) 
 GEOMETRIC_REPRESENTATION_ITEM ( )  RATIONAL_B_SPLINE_SURFACE ( (
 ( 1.000000000000000000, 0.4999999999999997224, 1.000000000000000000),
 ( 1.000000000000000000, 0.5048840838053595403, 1.000000000000000000),
 ( 1.000000000000000000, 0.5132072642500213888, 1.000000000000000000),
 ( 1.000000000000000000, 0.5290214861663711243, 1.000000000000000000),
 ( 1.000000000000000000, 0.5348648783786191796, 1.000000000000000000),
 ( 1.000000000000000000, 0.5473516051742142174, 1.000000000000000000),
 ( 1.000000000000000000, 0.5539126387906357918, 1.000000000000000000),
 ( 1.000000000000000000, 0.5674101295481593921, 1.000000000000000000),
 ( 1.000000000000000000, 0.5743474342084209372, 1.000000000000000000),
 ( 1.000000000000000000, 0.5883951384281623787, 1.000000000000000000),
 ( 1.000000000000000000, 0.5955302209471763364, 1.000000000000000000),
 ( 1.000000000000000000, 0.6167715304226695228, 1.000000000000000000),
 ( 1.000000000000000000, 0.6305661306848210357, 1.000000000000000000),
 ( 1.000000000000000000, 0.6565125894471607326, 1.000000000000000000),
 ( 1.000000000000000000, 0.6686743926051859077, 1.000000000000000000),
 ( 1.000000000000000000, 0.6851014456086408355, 1.000000000000000000),
 ( 1.000000000000000000, 0.6902475665164403695, 1.000000000000000000),
 ( 1.000000000000000000, 0.6997062435422888305, 1.000000000000000000),
 ( 1.000000000000000000, 0.7040363771866375853, 1.000000000000000000),
 ( 1.000000000000000000, 0.7157418617804421901, 1.000000000000000000),
 ( 1.000000000000000000, 0.7218341033859928535, 1.000000000000000000),
 ( 1.000000000000000000, 0.7280280015705831165, 1.000000000000000000),
 ( 1.000000000000000000, 0.7296036051598838723, 1.000000000000000000),
 ( 1.000000000000000000, 0.7316818214130017539, 1.000000000000000000),
 ( 1.000000000000000000, 0.7321927565546040295, 1.000000000000000000),
 ( 1.000000000000000000, 0.7321641879719948953, 1.000000000000000000),
 ( 1.000000000000000000, 0.7300624469253677029, 1.000000000000000000),
 ( 1.000000000000000000, 0.7238943330023113187, 1.000000000000000000),
 ( 1.000000000000000000, 0.7213359435419863797, 1.000000000000000000),
 ( 1.000000000000000000, 0.7152343487863939142, 1.000000000000000000),
 ( 1.000000000000000000, 0.7117056589944237288, 1.000000000000000000),
 ( 1.000000000000000000, 0.6999072021060018800, 1.000000000000000000),
 ( 1.000000000000000000, 0.6903911339382012846, 1.000000000000000000),
 ( 1.000000000000000000, 0.6741089150890702264, 1.000000000000000000),
 ( 1.000000000000000000, 0.6683461163768288360, 1.000000000000000000),
 ( 1.000000000000000000, 0.6562237482357344831, 1.000000000000000000),
 ( 1.000000000000000000, 0.6498375142660873793, 1.000000000000000000),
 ( 1.000000000000000000, 0.6302143011361827085, 1.000000000000000000),
 ( 1.000000000000000000, 0.6164540672887562911, 1.000000000000000000),
 ( 1.000000000000000000, 0.5885848209491306715, 1.000000000000000000),
 ( 1.000000000000000000, 0.5744580946949985334, 1.000000000000000000),
 ( 1.000000000000000000, 0.5540565490002123950, 1.000000000000000000),
 ( 1.000000000000000000, 0.5474350731751959076, 1.000000000000000000),
 ( 1.000000000000000000, 0.5350293539659718434, 1.000000000000000000),
 ( 1.000000000000000000, 0.5292092555093077522, 1.000000000000000000),
 ( 1.000000000000000000, 0.5186171472262492976, 1.000000000000000000),
 ( 1.000000000000000000, 0.5138445523878416576, 1.000000000000000000),
 ( 1.000000000000000000, 0.5056909436241932010, 1.000000000000000000),
 ( 1.000000000000000000, 0.5023956439952826925, 1.000000000000000000),
 ( 1.000000000000000000, 0.4999999999999995004, 1.000000000000000000) ) ) 
 REPRESENTATION_ITEM ( '' )  SURFACE ( )  );
#43720=ORIENTED_EDGE ( 'NONE', *, *, #64449, .T. ) ;
#43729=ORIENTED_EDGE ( 'NONE', *, *, #61088, .F. ) ;
#43737=CARTESIAN_POINT ( 'NONE',  ( -5.808548865027071351, -28.57390223679936980, 12.95295593664479483 ) ) ;
#43795=CARTESIAN_POINT ( 'NONE',  ( 2.990024434114437302, -31.21813892570122206, -14.24440799104838717 ) ) ;
#43818=ORIENTED_EDGE ( 'NONE', *, *, #48029, .F. ) ;
#43845=CARTESIAN_POINT ( 'NONE',  ( -19.56743653832047158, -33.00000000000000000, -5.000000000000003553 ) ) ;
#43910=EDGE_LOOP ( 'NONE', ( #27150, #9641, #38014, #37076, #11086, #35957, #28590 ) ) ;
#43923=CARTESIAN_POINT ( 'NONE',  ( -14.82142464308680907, -33.91165328791170452, -8.853132628082329703 ) ) ;
#43947=FACE_OUTER_BOUND ( 'NONE', #28609, .T. ) ;
#43956=CARTESIAN_POINT ( 'NONE',  ( 16.79789036561810889, -29.41979974037718293, -9.796743230926868051 ) ) ;
#43972=PLANE ( 'NONE',  #39261 ) ;
#43993=EDGE_CURVE ( 'NONE', #51364, #38363, #39247, .T. ) ;
#44035=AXIS2_PLACEMENT_3D ( 'NONE', #36013, #61622, #45037 ) ;
#44071=CARTESIAN_POINT ( 'NONE',  ( -12.11665614333141505, -29.85821820039599928, 8.776459307919161290 ) ) ;
#44095=ORIENTED_EDGE ( 'NONE', *, *, #55509, .F. ) ;
#44112=CIRCLE ( 'NONE', #15443, 3.999999999999999556 ) ;
#44120=CARTESIAN_POINT ( 'NONE',  ( 0.8665813290829081916, -31.03691730605172694, -14.44326482629603881 ) ) ;
#44157=CARTESIAN_POINT ( 'NONE',  ( 0.000000000000000000, -45.00000000000000000, 0.000000000000000000 ) ) ;
#44174=FACE_OUTER_BOUND ( 'NONE', #54754, .T. ) ;
#44181=CIRCLE ( 'NONE', #65376, 3.000000000000001332 ) ;
#44193=LINE ( 'NONE', #44499, #65117 ) ;
#44239=CARTESIAN_POINT ( 'NONE',  ( -7.187257474343136998, -31.45475789300778047, -14.12255545930396394 ) ) ;
#44268=CARTESIAN_POINT ( 'NONE',  ( -17.77323790556440386, -29.67638950762373540, -8.606028548248501053 ) ) ;
#44360=EDGE_CURVE ( 'NONE', #15355, #22226, #42161, .T. ) ;
#44375=CARTESIAN_POINT ( 'NONE',  ( 1.845799476744150569, -28.15607794640468597, 13.84328548073729870 ) ) ;
#44393=CARTESIAN_POINT ( 'NONE',  ( 25.00000000000000355, -30.00000000000000000, -5.000000000000000888 ) ) ;
#44422=CARTESIAN_POINT ( 'NONE',  ( 5.911253750797971662, -28.27393032148221863, -11.47047724608643371 ) ) ;
#44495=EDGE_CURVE ( 'NONE', #26603, #18880, #57101, .T. ) ;
#44497=CARTESIAN_POINT ( 'NONE',  ( 0.000000000000000000, -33.00000000000000000, 0.000000000000000000 ) ) ;
#44499=CARTESIAN_POINT ( 'NONE',  ( -25.00000000000000355, -28.99999999999999645, -5.000000000000000888 ) ) ;
#44501=EDGE_CURVE ( 'NONE', #2269, #8147, #50044, .T. ) ;
#44530=CARTESIAN_POINT ( 'NONE',  ( -25.00000000000000355, -28.99999999999999645, 1.530808498934191521E-15 ) ) ;
#44571=CARTESIAN_POINT ( 'NONE',  ( -19.27703245284564915, -30.00000000000000711, 5.988254523999585466 ) ) ;
#44590=ORIENTED_EDGE ( 'NONE', *, *, #25301, .F. ) ;
#44610=CARTESIAN_POINT ( 'NONE',  ( -0.9057367950582522198, -28.12814853318315400, -13.89764383195144326 ) ) ;
#44643=ADVANCED_FACE ( 'NONE', ( #26736 ), #29368, .T. ) ;
#44658=CARTESIAN_POINT ( 'NONE',  ( 30.66651853351974211, -3.164325622109354086, -24.36290982288815243 ) ) ;
#44688=CARTESIAN_POINT ( 'NONE',  ( -37.25000000000000711, -27.21021009056489603, 4.499999999999997335 ) ) ;
#44702=CARTESIAN_POINT ( 'NONE',  ( -0.4406170177989196524, -30.53628804997674706, 15.30998899416534975 ) ) ;
#44725=DIRECTION ( 'NONE',  ( 1.000000000000000000, -0.000000000000000000, 0.000000000000000000 ) ) ;
#44760=CARTESIAN_POINT ( 'NONE',  ( 5.268658153349320195, -26.03085267760928545, -15.19911252589913886 ) ) ;
#44761=EDGE_LOOP ( 'NONE', ( #35193, #29420, #24640, #26299 ) ) ;
#44803=ORIENTED_EDGE ( 'NONE', *, *, #22438, .T. ) ;
#44814=ADVANCED_FACE ( 'NONE', ( #39654 ), #9373, .F. ) ;
#44843=CARTESIAN_POINT ( 'NONE',  ( 15.82795513634483875, -34.24358411257726686, -7.361295665690556156 ) ) ;
#44876=ORIENTED_EDGE ( 'NONE', *, *, #50067, .T. ) ;
#44883=CARTESIAN_POINT ( 'NONE',  ( 0.000000000000000000, -33.00000000000000000, 0.000000000000000000 ) ) ;
#44894=VERTEX_POINT ( 'NONE', #28263 ) ;
#44920=CARTESIAN_POINT ( 'NONE',  ( 3.527934398658590709, -26.69696348912970763, 16.00979375678724281 ) ) ;
#44929=CARTESIAN_POINT ( 'NONE',  ( -0.5028117989624658613, -26.55343892596427224, -16.22424428316958611 ) ) ;
#44963=CARTESIAN_POINT ( 'NONE',  ( -2.287538219536363382, -28.18941229671508708, -13.77533426008797335 ) ) ;
#45001=EDGE_CURVE ( 'NONE', #45854, #18262, #29194, .T. ) ;
#45011=CARTESIAN_POINT ( 'NONE',  ( 49.78928762170308886, -0.04292493490551599344, 3.265281182697543638 ) ) ;
#45017=CARTESIAN_POINT ( 'NONE',  ( 6.333770985428929912, -31.24637718316046531, 14.41548832156072102 ) ) ;
#45019=AXIS2_PLACEMENT_3D ( 'NONE', #20295, #40572, #55878 ) ;
#45037=DIRECTION ( 'NONE',  ( 0.000000000000000000, 0.000000000000000000, 1.000000000000000000 ) ) ;
#45043=CARTESIAN_POINT ( 'NONE',  ( -13.20530710592869283, -34.09051099065911217, 9.405657446765959051 ) ) ;
#45045=CARTESIAN_POINT ( 'NONE',  ( -17.05023968204110929, -34.50000000000000000, -4.356789313881321846 ) ) ;
#45049=ORIENTED_EDGE ( 'NONE', *, *, #50357, .F. ) ;
#45055=CARTESIAN_POINT ( 'NONE',  ( 4.972137933590733638, -28.45452681573965137, 13.21946257705964811 ) ) ;
#45100=CARTESIAN_POINT ( 'NONE',  ( -14.83484859610164364, -34.67578963454042196, -7.338086519100818883 ) ) ;
#45107=CARTESIAN_POINT ( 'NONE',  ( 9.079541994506246994, -32.62122108031978485, -12.39463523794014321 ) ) ;
#45130=FILL_AREA_STYLE_COLOUR ( '', #42980 ) ;
#45131=LINE ( 'NONE', #65391, #65103 ) ;
#45149=CARTESIAN_POINT ( 'NONE',  ( 25.00000000000000355, -9.999999999999998224, 1.530808498934191521E-15 ) ) ;
#45185=CARTESIAN_POINT ( 'NONE',  ( -14.24371601685106548, -33.70914924250434552, 9.547107017906496296 ) ) ;
#45192=DIRECTION ( 'NONE',  ( 0.000000000000000000, 0.000000000000000000, 1.000000000000000000 ) ) ;
#45228=CARTESIAN_POINT ( 'NONE',  ( 17.99690872998901980, -28.74566129397116754, 8.126501682513223912 ) ) ;
#45250=FILL_AREA_STYLE ('',( #24977 ) ) ;
#45289=CARTESIAN_POINT ( 'NONE',  ( 0.9185403246812442468, -30.53691730605505228, -15.30924831176142042 ) ) ;
#45304=DIRECTION ( 'NONE',  ( 0.000000000000000000, 1.000000000000000000, 0.000000000000000000 ) ) ;
#45331=CARTESIAN_POINT ( 'NONE',  ( 37.50900221036943805, -2.222235401316472903, 21.66089349574500744 ) ) ;
#45333=CARTESIAN_POINT ( 'NONE',  ( -28.29050403390679591, -3.446535021889315598, -24.79622249374515519 ) ) ;
#45371=CARTESIAN_POINT ( 'NONE',  ( 8.372133460183182052, -31.76502814486162407, 13.66429824708607477 ) ) ;
#45373=DIRECTION ( 'NONE',  ( -0.9688695217174486674, 0.000000000000000000, -0.2475719085175094036 ) ) ;
#45381=EDGE_LOOP ( 'NONE', ( #34081, #14963, #40492, #43402 ) ) ;
#45415=CARTESIAN_POINT ( 'NONE',  ( 8.088853370213684002, -28.65367229866794219, -10.33367282332731385 ) ) ;
#45429=FACE_OUTER_BOUND ( 'NONE', #31341, .T. ) ;
#45431=CARTESIAN_POINT ( 'NONE',  ( -22.00000000000000711, -20.00000000000000000, 2.449293598294706907E-15 ) ) ;
#45455=B_SPLINE_CURVE_WITH_KNOTS ( 'NONE', 3,
 ( #31272, #57203, #40919, #30927, #36902, #21949, #36585, #51574, #50899, #26936, #47236, #46556, #62180, #5349, #1350, #1013, #56888, #21279, #11313, #25963, #41555, #11629, #20947, #1683, #31899, #31580, #16632, #51888, #690, #15315, #52221, #41225, #35591, #6332, #46248, #26598, #46890, #10316, #38545, #42872, #63160, #63797, #17626, #27921, #53188, #48229 ),
 .UNSPECIFIED., .F., .F.,
 ( 4, 2, 2, 2, 2, 2, 2, 2, 2, 2, 2, 2, 2, 2, 2, 2, 2, 2, 2, 2, 2, 2, 4 ),
 ( 0.000000000000000000, 0.001519118309396224427, 0.003038236618792448853, 0.004557354928188673063, 0.006076473237584897706, 0.009114709856377337452, 0.01215294647516977807, 0.01519118309396221868, 0.01822941971275466103, 0.01974853802215088133, 0.02126765633154709817, 0.02430589295033953531, 0.02582501125973575562, 0.02734412956913197593, 0.03038236618792440960, 0.03342060280671684674, 0.03645883942550928736, 0.03949707604430172797, 0.04101619435369794481, 0.04253531266309416164, 0.04405443097249037848, 0.04557354928188660226, 0.04861178590067902899 ),
 .UNSPECIFIED. ) ;
#45484=EDGE_CURVE ( 'NONE', #18262, #30237, #48512, .T. ) ;
#45501=CIRCLE ( 'NONE', #60363, 19.99999999999999645 ) ;
#45532=AXIS2_PLACEMENT_3D ( 'NONE', #43845, #54152, #63144 ) ;
#45535=FACE_OUTER_BOUND ( 'NONE', #59966, .T. ) ;
#45564=DIRECTION ( 'NONE',  ( 0.000000000000000000, -1.000000000000000000, 0.000000000000000000 ) ) ;
#45587=EDGE_LOOP ( 'NONE', ( #9299, #16721, #44095, #54632, #5575, #52193, #55360 ) ) ;
#45588=DIRECTION ( 'NONE',  ( 1.000000000000000000, -0.000000000000000000, -0.000000000000000000 ) ) ;
#45606=CARTESIAN_POINT ( 'NONE',  ( -6.246056400524260255, -31.23659747722423319, -14.42616998329098799 ) ) ;
#45617=CARTESIAN_POINT ( 'NONE',  ( -0.8753493882091067935, -31.04850208196501526, 14.43082775300658938 ) ) ;
#45657=CARTESIAN_POINT ( 'NONE',  ( 47.41971561978370886, -0.5128904950765936777, 11.09198065024578916 ) ) ;
#45660=CARTESIAN_POINT ( 'NONE',  ( -25.82596324657533415, -3.714872568654937091, -25.00000000000000355 ) ) ;
#45688=CARTESIAN_POINT ( 'NONE',  ( -12.89187373143239945, -27.44222185127960145, 12.55025375818352629 ) ) ;
#45699=CARTESIAN_POINT ( 'NONE',  ( 15.30590914263659386, -29.00884126188377365, 11.24874127360776654 ) ) ;
#45729=EDGE_CURVE ( 'NONE', #26969, #45854, #24715, .T. ) ;
#45732=EDGE_CURVE ( 'NONE', #659, #26603, #4934, .T. ) ;
#45751=CARTESIAN_POINT ( 'NONE',  ( 18.18435566811206527, -28.78814669831782780, -7.856426167042674713 ) ) ;
#45769=DIRECTION ( 'NONE',  ( -1.000000000000000000, -0.000000000000000000, -0.000000000000000000 ) ) ;
#45795=ORIENTED_EDGE ( 'NONE', *, *, #13158, .F. ) ;
#45851=ORIENTED_EDGE ( 'NONE', *, *, #3123, .T. ) ;
#45854=VERTEX_POINT ( 'NONE', #42499 ) ;
#45880=AXIS2_PLACEMENT_3D ( 'NONE', #30973, #40959, #34960 ) ;
#45887=CIRCLE ( 'NONE', #22474, 3.999999999999999112 ) ;
#45891=CARTESIAN_POINT ( 'NONE',  ( 18.54281746013980126, -28.86505449477128593, 7.298814700743933237 ) ) ;
#45899=CARTESIAN_POINT ( 'NONE',  ( 37.25000000000000711, -20.00000000000000000, 2.449293598294706907E-15 ) ) ;
#45930=EDGE_CURVE ( 'NONE', #52466, #49767, #33682, .T. ) ;
#45940=EDGE_LOOP ( 'NONE', ( #31813, #1346, #35369, #58641 ) ) ;
#45957=CARTESIAN_POINT ( 'NONE',  ( -8.789023433376842220, -31.87591480792562137, -13.49878314047872507 ) ) ;
#46049=CARTESIAN_POINT ( 'NONE',  ( 8.782331025771487276, -31.88110954670732866, 13.48440172003490289 ) ) ;
#46092=CARTESIAN_POINT ( 'NONE',  ( 14.33157020396088832, -34.50275931095601578, 8.076358832431466794 ) ) ;
#46095=CARTESIAN_POINT ( 'NONE',  ( -6.824045466202398380, -31.96248520358999201, -13.34027024243112791 ) ) ;
#46102=CARTESIAN_POINT ( 'NONE',  ( 11.58535936493820273, -27.13779202276463920, -13.20710129366601926 ) ) ;
#46149=ORIENTED_EDGE ( 'NONE', *, *, #63940, .T. ) ;
#46210=EDGE_CURVE ( 'NONE', #31440, #30237, #63055, .T. ) ;
#46211=CARTESIAN_POINT ( 'NONE',  ( -16.47895549814540672, -34.42947327577542893, 6.127516784536641836 ) ) ;
#46216=CARTESIAN_POINT ( 'NONE',  ( -40.83349710434619340, -1.696348104764183962, -18.10529304745324097 ) ) ;
#46247=CARTESIAN_POINT ( 'NONE',  ( -41.00000000000000711, -25.03188948156373073, -4.500000000000008882 ) ) ;
#46248=CARTESIAN_POINT ( 'NONE',  ( -13.26546321032139986, -27.53582555932707976, -12.33704161722047488 ) ) ;
#46249=CARTESIAN_POINT ( 'NONE',  ( 5.527856869237428583, -26.90719658711817885, 15.68471180892751526 ) ) ;
#46271=CARTESIAN_POINT ( 'NONE',  ( 48.45393016956177945, -0.3105270330721123240, -5.105971556042214310 ) ) ;
#46275=ORIENTED_EDGE ( 'NONE', *, *, #5727, .F. ) ;
#46286=CARTESIAN_POINT ( 'NONE',  ( 13.26995653566893019, -33.36016745060648958, -10.56634385159335388 ) ) ;
#46295=CARTESIAN_POINT ( 'NONE',  ( -7.228961821822758260, -32.07041743672118628, 13.19626196499948634 ) ) ;
#46329=CARTESIAN_POINT ( 'NONE',  ( 47.76247274761329464, -0.4463159248369739651, -10.36992351718251015 ) ) ;
#46357=CARTESIAN_POINT ( 'NONE',  ( 5.268658153349320195, -26.03085267760928545, 15.19911252589913886 ) ) ;
#46367=CARTESIAN_POINT ( 'NONE',  ( 3.643024398545848808, -28.29981509102552550, 13.54931501599828358 ) ) ;
#46403=AXIS2_PLACEMENT_3D ( 'NONE', #16998, #6718, #47597 ) ;
#46412=CARTESIAN_POINT ( 'NONE',  ( 8.309432179406254448, -32.38110954670829500, -12.75850010368669629 ) ) ;
#46516=CARTESIAN_POINT ( 'NONE',  ( 41.00000000000000000, -25.34319448863032065, -3.012683490291701016 ) ) ;
#46517=CARTESIAN_POINT ( 'NONE',  ( -17.05023968204110574, -34.50000000000000000, 4.356789313881320957 ) ) ;
#46520=CARTESIAN_POINT ( 'NONE',  ( -12.11665614333000462, -29.85821820039411278, -8.776459307919635577 ) ) ;
#46525=ORIENTED_EDGE ( 'NONE', *, *, #14446, .T. ) ;
#46541=CARTESIAN_POINT ( 'NONE',  ( 4.308196110052892319E-12, -30.53649492335491189, 15.30974548841782656 ) ) ;
#46556=CARTESIAN_POINT ( 'NONE',  ( 13.26780778037858433, -27.53645921949369679, -12.33502842928022325 ) ) ;
#46557=DIRECTION ( 'NONE',  ( -0.2475719085175098477, 0.000000000000000000, -0.9688695217174486674 ) ) ;
#46581=CARTESIAN_POINT ( 'NONE',  ( 47.77118093457289660, -0.4451837999798747281, 7.743266003128067787 ) ) ;
#46598=CARTESIAN_POINT ( 'NONE',  ( 8.617947477505378373, -29.08580380500674778, -11.66524603227210122 ) ) ;
#46642=DIRECTION ( 'NONE',  ( 1.826024711554533420E-16, 0.000000000000000000, -1.000000000000000000 ) ) ;
#46675=CARTESIAN_POINT ( 'NONE',  ( 2.128776824815522772, -25.76454106360162299, 15.60647423695309222 ) ) ;
#46704=DIRECTION ( 'NONE',  ( 0.000000000000000000, 1.000000000000000000, 0.000000000000000000 ) ) ;
#46743=COLOUR_RGB ( '', 0.31764706, 0.68627451, 0.89019608) ;
#46760=CARTESIAN_POINT ( 'NONE',  ( -25.00000000000000355, -9.999999999999998224, 5.000000000000000888 ) ) ;
#46765=CIRCLE ( 'NONE', #10632, 1.500000000000000222 ) ;
#46772=EDGE_LOOP ( 'NONE', ( #27718, #53119 ) ) ;
#46793=CIRCLE ( 'NONE', #38288, 17.59807621135332312 ) ;
#46796=CARTESIAN_POINT ( 'NONE',  ( 25.00000000000000355, -9.999999999999998224, -25.00000000000000000 ) ) ;
#46890=CARTESIAN_POINT ( 'NONE',  ( -14.88966238093840744, -27.95127710492162620, -11.23339344092910252 ) ) ;
#46918=CARTESIAN_POINT ( 'NONE',  ( 48.68114316863541546, -0.2655233219083136254, 3.919294168552611257 ) ) ;
#46934=CARTESIAN_POINT ( 'NONE',  ( 14.48396081724352769, -30.02861890643281839, -3.972401191364113515 ) ) ;
#46943=CARTESIAN_POINT ( 'NONE',  ( -11.32744364968265138, -33.39367328239647748, 11.05351320890950362 ) ) ;
#46975=DIRECTION ( 'NONE',  ( 0.000000000000000000, -1.000000000000000000, 0.000000000000000000 ) ) ;
#46997=VERTEX_POINT ( 'NONE', #21702 ) ;
#47021=CARTESIAN_POINT ( 'NONE',  ( -0.4223990570890304164, -27.81390085543024426, 12.58355210400704394 ) ) ;
#47122=CYLINDRICAL_SURFACE ( 'NONE', #38509, 25.00000000000000000 ) ;
#47161=CARTESIAN_POINT ( 'NONE',  ( -33.02316666837518255, -2.861627175174543680, 23.69173491641419105 ) ) ;
#47178=ORIENTED_EDGE ( 'NONE', *, *, #1799, .T. ) ;
#47216=DIRECTION ( 'NONE',  ( -1.000000000000000000, -0.000000000000000000, -0.000000000000000000 ) ) ;
#47236=CARTESIAN_POINT ( 'NONE',  ( 14.88292245651501666, -27.94758995389113210, -11.26211297105861142 ) ) ;
#47243=LINE ( 'NONE', #6337, #41947 ) ;
#47249=AXIS2_PLACEMENT_3D ( 'NONE', #39762, #60054, #25129 ) ;
#47261=CARTESIAN_POINT ( 'NONE',  ( 48.79774903324594248, -0.2423453535664415182, 3.134413741627073868 ) ) ;
#47273=CARTESIAN_POINT ( 'NONE',  ( 37.25000000000000711, -27.32965888902624840, 3.759436751556509915 ) ) ;
#47277=CARTESIAN_POINT ( 'NONE',  ( 13.56792483472022681, -30.10715271124523440, -6.611461891173261662 ) ) ;
#47285=CARTESIAN_POINT ( 'NONE',  ( 15.04427341496945481, -34.74416750921023578, -6.992747701485109602 ) ) ;
#47309=PLANE ( 'NONE',  #54016 ) ;
#47320=DIRECTION ( 'NONE',  ( 0.000000000000000000, 0.000000000000000000, 1.000000000000000000 ) ) ;
#47324=DIRECTION ( 'NONE',  ( -1.000000000000000000, 0.000000000000000000, 0.000000000000000000 ) ) ;
#47349=ORIENTED_EDGE ( 'NONE', *, *, #11023, .T. ) ;
#47351=CARTESIAN_POINT ( 'NONE',  ( 4.682340427901537261, -31.48164499408211014, 13.94155213824621953 ) ) ;
#47373=EDGE_LOOP ( 'NONE', ( #36329, #55417, #52718, #22401, #47349, #5957, #47431 ) ) ;
#47409=FACE_OUTER_BOUND ( 'NONE', #14453, .T. ) ;
#47426=AXIS2_PLACEMENT_3D ( 'NONE', #24319, #34297, #8717 ) ;
#47431=ORIENTED_EDGE ( 'NONE', *, *, #7305, .T. ) ;
#47438=CARTESIAN_POINT ( 'NONE',  ( -38.94999461337798152, -1.999059167504504630, 19.54503265464386885 ) ) ;
#47483=CARTESIAN_POINT ( 'NONE',  ( -15.66605021877826331, -34.92947327577397942, -5.825441821991796942 ) ) ;
#47548=CARTESIAN_POINT ( 'NONE',  ( 15.74859868605385138, -29.13321728093752938, 10.87107032828077102 ) ) ;
#47567=CARTESIAN_POINT ( 'NONE',  ( 25.00000000000000355, -3.797884998337192286, 23.99999999999999289 ) ) ;
#47585=CARTESIAN_POINT ( 'NONE',  ( 9.730232070128620236, -27.62176360438186506, -14.46115055101679125 ) ) ;
#47597=DIRECTION ( 'NONE',  ( 0.000000000000000000, 0.000000000000000000, -1.000000000000000000 ) ) ;
#47654=DIRECTION ( 'NONE',  ( -1.000000000000000000, 0.000000000000000000, 0.000000000000000000 ) ) ;
#47662=CARTESIAN_POINT ( 'NONE',  ( 10.51584247049436449, -29.12274881419789807, 8.353506175201449224 ) ) ;
#47751=CARTESIAN_POINT ( 'NONE',  ( -18.19295774167957092, -29.77901320112238892, 7.993354913176278664 ) ) ;
#47754=CARTESIAN_POINT ( 'NONE',  ( -45.37278721346743282, -0.8995687559121183785, -12.71067884230443923 ) ) ;
#47796=CARTESIAN_POINT ( 'NONE',  ( -36.06679944573490104, -2.440416481716451091, 22.47657575504853256 ) ) ;
#47890=CARTESIAN_POINT ( 'NONE',  ( -4.578562111148198888, -30.90741127680383471, 14.86059354493743179 ) ) ;
#47891=TOROIDAL_SURFACE ( 'NONE', #4427, 5.000000000000000888, 20.00000000000000000 ) ;
#47927=CARTESIAN_POINT ( 'NONE',  ( 3.474089039505902754, -31.27092243478551126, -14.18576039181806614 ) ) ;
#47961=AXIS2_PLACEMENT_3D ( 'NONE', #30205, #20561, #49834 ) ;
#47965=AXIS2_PLACEMENT_3D ( 'NONE', #48005, #11742, #37350 ) ;
#47970=CARTESIAN_POINT ( 'NONE',  ( 22.00000000000000711, -20.00000000000000000, 2.449293598294706907E-15 ) ) ;
#48001=CARTESIAN_POINT ( 'NONE',  ( 16.21117406328132304, -34.99999999999999289, 4.142385751841744401 ) ) ;
#48005=CARTESIAN_POINT ( 'NONE',  ( -25.00000000000000355, -9.999999999999998224, 5.000000000000000888 ) ) ;
#48019=VERTEX_POINT ( 'NONE', #20720 ) ;
#48029=EDGE_CURVE ( 'NONE', #57274, #43036, #30719, .T. ) ;
#48036=CIRCLE ( 'NONE', #27854, 24.00000000000000000 ) ;
#48094=CARTESIAN_POINT ( 'NONE',  ( -17.34314652423584491, -29.56569286319672685, 9.163921882790974749 ) ) ;
#48097=CARTESIAN_POINT ( 'NONE',  ( -49.00067463083242103, -0.2018647702350209738, -0.7653472444253763829 ) ) ;
#48153=AXIS2_PLACEMENT_3D ( 'NONE', #59558, #9647, #24973 ) ;
#48154=FACE_OUTER_BOUND ( 'NONE', #47373, .T. ) ;
#48167=DIRECTION ( 'NONE',  ( -0.9688695217174487784, 0.000000000000000000, -0.2475719085175095702 ) ) ;
#48215=DIRECTION ( 'NONE',  ( -1.000000000000000000, -0.000000000000000000, -0.000000000000000000 ) ) ;
#48229=CARTESIAN_POINT ( 'NONE',  ( -19.56743653832046803, -28.99999999999999645, -4.999999999999997335 ) ) ;
#48235=ORIENTED_EDGE ( 'NONE', *, *, #61088, .T. ) ;
#48239=CARTESIAN_POINT ( 'NONE',  ( 22.00000000000000711, -20.00000000000000000, 2.449293598294706907E-15 ) ) ;
#48249=EDGE_CURVE ( 'NONE', #56931, #3747, #20104, .T. ) ;
#48258=CARTESIAN_POINT ( 'NONE',  ( 37.00843563923471180, -2.297594674915183877, 20.79457751400812882 ) ) ;
#48272=DIRECTION ( 'NONE',  ( 0.000000000000000000, 1.000000000000000000, 0.000000000000000000 ) ) ;
#48283=CARTESIAN_POINT ( 'NONE',  ( 15.63877597542558107, -34.91516792956247173, -5.826750174076742006 ) ) ;
#48320=ADVANCED_FACE ( 'NONE', ( #57497 ), #42691, .F. ) ;
#48322=ORIENTED_EDGE ( 'NONE', *, *, #45729, .T. ) ;
#48331=STYLED_ITEM ( 'NONE', ( #49790 ), #4012 ) ;
#48346=CARTESIAN_POINT ( 'NONE',  ( 16.10228578084485562, -34.99999999976227372, 4.568518662555822729 ) ) ;
#48366=EDGE_CURVE ( 'NONE', #51562, #26969, #33906, .T. ) ;
#48400=DIRECTION ( 'NONE',  ( -1.000000000000000000, 0.000000000000000000, 0.000000000000000000 ) ) ;
#48423=CARTESIAN_POINT ( 'NONE',  ( -12.36714175812590355, -29.91041276695339590, 8.471522614801738627 ) ) ;
#48449=CARTESIAN_POINT ( 'NONE',  ( -25.00000000000000355, -3.797884998337192286, -24.99999999999999289 ) ) ;
#48512=CIRCLE ( 'NONE', #46403, 23.66025403784440329 ) ;
#48533=ADVANCED_FACE ( 'NONE', ( #13955 ), #20146, .T. ) ;
#48549=CARTESIAN_POINT ( 'NONE',  ( 6.333770985417318755, -31.24637718315787183, -14.41548832156423998 ) ) ;
#48558=ADVANCED_FACE ( 'NONE', ( #65161 ), #43535, .T. ) ;
#48567=CARTESIAN_POINT ( 'NONE',  ( 28.93866847389637798, -3.371687389997651163, 23.68754010782029695 ) ) ;
#48593=CARTESIAN_POINT ( 'NONE',  ( -19.26763262626407069, -29.00000000000000000, 5.969230316860641317 ) ) ;
#48641=FACE_BOUND ( 'NONE', #57439, .T. ) ;
#48645=ORIENTED_EDGE ( 'NONE', *, *, #48366, .T. ) ;
#48742=CARTESIAN_POINT ( 'NONE',  ( 0.9290584433855317847, -28.11997881881914196, 13.91374373156083166 ) ) ;
#48758=DIRECTION ( 'NONE',  ( -1.000000000000000000, -0.000000000000000000, -0.000000000000000000 ) ) ;
#48779=DIRECTION ( 'NONE',  ( 1.000000000000000000, 0.000000000000000000, 0.000000000000000000 ) ) ;
#48792=EDGE_CURVE ( 'NONE', #659, #40350, #63703, .T. ) ;
#48797=CARTESIAN_POINT ( 'NONE',  ( 4.225235259830817824, -25.92188032005471143, -15.36840686706593928 ) ) ;
#48806=EDGE_CURVE ( 'NONE', #37781, #34941, #41393, .T. ) ;
#48858=AXIS2_PLACEMENT_3D ( 'NONE', #61413, #30503, #10542 ) ;
#48925=CARTESIAN_POINT ( 'NONE',  ( -13.93947072118801600, -33.60066931048471872, -9.878030726373578929 ) ) ;
#48930=VECTOR ( 'NONE', #3223, 1000.000000000000000 ) ;
#48955=AXIS2_PLACEMENT_3D ( 'NONE', #36447, #52073, #7159 ) ;
#48978=DIRECTION ( 'NONE',  ( 0.000000000000000000, 0.000000000000000000, 1.000000000000000000 ) ) ;
#48979=EDGE_LOOP ( 'NONE', ( #4586, #12840, #46525, #61171 ) ) ;
#49073=DIRECTION ( 'NONE',  ( 0.000000000000000000, 1.000000000000000000, 0.000000000000000000 ) ) ;
#49085=CARTESIAN_POINT ( 'NONE',  ( -12.82483530079774603, -29.99871789793389709, 7.856364084351554311 ) ) ;
#49090=ORIENTED_EDGE ( 'NONE', *, *, #58494, .T. ) ;
#49135=CARTESIAN_POINT ( 'NONE',  ( -2.167161191928854258, -27.87656208324061069, -12.44306432472098756 ) ) ;
#49154=LINE ( 'NONE', #65701, #20177 ) ;
#49159=FILL_AREA_STYLE ('',( #45130 ) ) ;
#49174=PLANE ( 'NONE',  #54429 ) ;
#49215=CARTESIAN_POINT ( 'NONE',  ( 13.92922077006575599, -33.59874296436084506, -9.921733781854390699 ) ) ;
#49224=CARTESIAN_POINT ( 'NONE',  ( -7.187257474332334972, -31.45475789300513370, 14.12255545930775469 ) ) ;
#49242=ADVANCED_FACE ( 'NONE', ( #35313 ), #35643, .F. ) ;
#49255=DIRECTION ( 'NONE',  ( -1.000000000000000000, -0.000000000000000000, -0.000000000000000000 ) ) ;
#49305=PRODUCT ( 'Inner cradle housing', 'Inner cradle housing', '', ( #17497 ) ) ;
#49334=CARTESIAN_POINT ( 'NONE',  ( 19.43600575278776788, -28.99999999999999289, 5.424900065531946147 ) ) ;
#49412=DIRECTION ( 'NONE',  ( -1.000000000000000000, -0.000000000000000000, -0.000000000000000000 ) ) ;
#49419=CARTESIAN_POINT ( 'NONE',  ( 0.9185403246812403610, -30.53691730605505228, 15.30924831176142042 ) ) ;
#49447=EDGE_CURVE ( 'NONE', #11603, #30420, #1172, .T. ) ;
#49463=CARTESIAN_POINT ( 'NONE',  ( -7.278994278378053018, -26.30414574191657096, -14.75709246356266036 ) ) ;
#49484=SURFACE_STYLE_FILL_AREA ( #49159 ) ;
#49497=FACE_OUTER_BOUND ( 'NONE', #65164, .T. ) ;
#49532=CARTESIAN_POINT ( 'NONE',  ( 13.29259107886408131, -33.36832009551300615, -10.54479676546161926 ) ) ;
#49583=CARTESIAN_POINT ( 'NONE',  ( 39.82770826892757299, -25.90431001312668968, 4.499999999999997335 ) ) ;
#49612=ADVANCED_FACE ( 'NONE', ( #40561, #4347 ), #24956, .F. ) ;
#49637=CARTESIAN_POINT ( 'NONE',  ( -8.269707202464296358, -27.33416996378218755, -14.97774446421700922 ) ) ;
#49672=ORIENTED_EDGE ( 'NONE', *, *, #25939, .T. ) ;
#49704=DIRECTION ( 'NONE',  ( 0.000000000000000000, 1.000000000000000000, 0.000000000000000000 ) ) ;
#49707=CARTESIAN_POINT ( 'NONE',  ( -12.19463663866909187, -29.31670792731426545, 5.824636309908064469 ) ) ;
#49719=CARTESIAN_POINT ( 'NONE',  ( -11.87635721006996192, -32.86858074101603222, 11.71246211286135619 ) ) ;
#49732=EDGE_LOOP ( 'NONE', ( #23861, #4641 ) ) ;
#49745=EDGE_CURVE ( 'NONE', #53403, #18319, #63806, .T. ) ;
#49759=CARTESIAN_POINT ( 'NONE',  ( -16.21117406328131949, -35.00000000000000000, -4.142385751841763053 ) ) ;
#49766=CARTESIAN_POINT ( 'NONE',  ( -4.291397156012838110, -28.05769852054764968, -12.02237517917411047 ) ) ;
#49767=VERTEX_POINT ( 'NONE', #27556 ) ;
#49782=LINE ( 'NONE', #4231, #65149 ) ;
#49785=DIRECTION ( 'NONE',  ( 0.000000000000000000, 1.000000000000000000, 0.000000000000000000 ) ) ;
#49790=PRESENTATION_STYLE_ASSIGNMENT (( #24184 ) ) ;
#49795=DIRECTION ( 'NONE',  ( -1.000000000000000000, 0.000000000000000000, 0.000000000000000000 ) ) ;
#49834=DIRECTION ( 'NONE',  ( 0.000000000000000000, 0.000000000000000000, 1.000000000000000000 ) ) ;
#49888=PLANE ( 'NONE',  #54976 ) ;
#49893=CARTESIAN_POINT ( 'NONE',  ( -13.30196514322741841, -33.37310655729432085, -10.51054543287389542 ) ) ;
#49894=CIRCLE ( 'NONE', #50934, 22.50555349946515449 ) ;
#49909=ORIENTED_EDGE ( 'NONE', *, *, #64449, .F. ) ;
#49918=CARTESIAN_POINT ( 'NONE',  ( -15.75855542457932046, -29.13485235466247403, 10.82860303369087873 ) ) ;
#49948=EDGE_LOOP ( 'NONE', ( #61297, #43720, #64738, #39478 ) ) ;
#49956=CARTESIAN_POINT ( 'NONE',  ( 4.532733354134117931, -28.39821948934984874, -13.34103783736786042 ) ) ;
#49965=DIRECTION ( 'NONE',  ( 0.000000000000000000, 0.000000000000000000, 1.000000000000000000 ) ) ;
#49991=ADVANCED_FACE ( 'NONE', ( #4261 ), #60688, .F. ) ;
#50006=CARTESIAN_POINT ( 'NONE',  ( -47.77550903397568760, -0.4437794964969083433, -10.34167951973068611 ) ) ;
#50009=CARTESIAN_POINT ( 'NONE',  ( 3.202861212859688056, -30.72210164159773882, 15.08749394223661788 ) ) ;
#50035=CARTESIAN_POINT ( 'NONE',  ( -18.19295774167957447, -28.79006254106626272, 7.843687167517533254 ) ) ;
#50044=LINE ( 'NONE', #14443, #36866 ) ;
#50045=CIRCLE ( 'NONE', #4390, 3.000000000000000444 ) ;
#50046=CARTESIAN_POINT ( 'NONE',  ( 13.85759530760384628, -30.12605952702068279, 5.992721990255546416 ) ) ;
#50067=EDGE_CURVE ( 'NONE', #30237, #18262, #31996, .T. ) ;
#50074=ADVANCED_FACE ( 'NONE', ( #16196 ), #5924, .T. ) ;
#50096=CARTESIAN_POINT ( 'NONE',  ( -15.99047871552766331, -35.00000000000001421, -5.006074194136237665 ) ) ;
#50101=CARTESIAN_POINT ( 'NONE',  ( 3.413903065650966351, -31.27385512440588400, -14.18194743136197289 ) ) ;
#50120=CARTESIAN_POINT ( 'NONE',  ( 19.56743653832047514, -28.99999999999999645, 4.999999999999997335 ) ) ;
#50125=( LENGTH_UNIT ( ) NAMED_UNIT ( * ) SI_UNIT ( .MILLI., .METRE. ) );
#50127=DIRECTION ( 'NONE',  ( -0.000000000000000000, 1.000000000000000000, 0.000000000000000000 ) ) ;
#50148=FACE_BOUND ( 'NONE', #64635, .T. ) ;
#50154=CIRCLE ( 'NONE', #24656, 1.500000000000000444 ) ;
#50218=ORIENTED_EDGE ( 'NONE', *, *, #54229, .T. ) ;
#50229=AXIS2_PLACEMENT_3D ( 'NONE', #57714, #26448, #12136 ) ;
#50235=CARTESIAN_POINT ( 'NONE',  ( -9.737135312703241397, -26.73636926326595642, 14.00099174170044058 ) ) ;
#50249=EDGE_CURVE ( 'NONE', #3889, #43541, #12868, .T. ) ;
#50267=CARTESIAN_POINT ( 'NONE',  ( -19.27703245284566691, -30.00000000000001066, -5.988254523999591683 ) ) ;
#50278=ORIENTED_EDGE ( 'NONE', *, *, #7305, .F. ) ;
#50302=CARTESIAN_POINT ( 'NONE',  ( -5.261125060310215318, -26.86576352283318059, -15.75274798952653832 ) ) ;
#50349=CARTESIAN_POINT ( 'NONE',  ( 36.06592381555555704, -2.436921198044744497, 22.43244911821615162 ) ) ;
#50352=CARTESIAN_POINT ( 'NONE',  ( -49.78928762170311018, -0.04292493490549997154, -3.265281182697543638 ) ) ;
#50357=EDGE_CURVE ( 'NONE', #40350, #54896, #45887, .T. ) ;
#50378=CARTESIAN_POINT ( 'NONE',  ( -14.91771861688918399, -27.95837112815216230, 11.21176701200369763 ) ) ;
#50390=CARTESIAN_POINT ( 'NONE',  ( 12.84304429912246981, -30.00680403999870194, 7.859709520792756088 ) ) ;
#50410=DIRECTION ( 'NONE',  ( 0.000000000000000000, 0.000000000000000000, 1.000000000000000000 ) ) ;
#50435=CARTESIAN_POINT ( 'NONE',  ( 17.33919137821584044, -28.58640580301184286, -8.960163943132222641 ) ) ;
#50453=EDGE_CURVE ( 'NONE', #18319, #14466, #39086, .T. ) ;
#50464=DIRECTION ( 'NONE',  ( 0.000000000000000000, 0.000000000000000000, 1.000000000000000000 ) ) ;
#50483=CARTESIAN_POINT ( 'NONE',  ( 22.00000000000000711, -20.00000000000000000, 1.500000000000002887 ) ) ;
#50560=CARTESIAN_POINT ( 'NONE',  ( -7.856485614137364237, -26.39148214816155757, 14.61473980079826518 ) ) ;
#50567=ADVANCED_FACE ( 'NONE', ( #31417 ), #51717, .T. ) ;
#50593=CARTESIAN_POINT ( 'NONE',  ( -2.534465382079153173, -26.62629929685681063, -16.11622222973024421 ) ) ;
#50620=CARTESIAN_POINT ( 'NONE',  ( 5.268658153348980910, -26.87458176590483916, -15.73590792199858868 ) ) ;
#50643=ORIENTED_EDGE ( 'NONE', *, *, #45001, .T. ) ;
#50644=LINE ( 'NONE', #55633, #63558 ) ;
#50665=CARTESIAN_POINT ( 'NONE',  ( 28.29050403390680302, -3.446535021889316930, 24.79622249374515519 ) ) ;
#50667=CARTESIAN_POINT ( 'NONE',  ( -40.23304019309010471, -1.796181362175412133, -19.88949158386754235 ) ) ;
#50670=CARTESIAN_POINT ( 'NONE',  ( 1.836544102203957696, -30.58412608844328417, 15.25442441212345557 ) ) ;
#50686=AXIS2_PLACEMENT_3D ( 'NONE', #32855, #12922, #58839 ) ;
#50696=CARTESIAN_POINT ( 'NONE',  ( -12.58062741647496274, -29.25281707778071549, 4.759732266940784662 ) ) ;
#50706=CARTESIAN_POINT ( 'NONE',  ( 6.272189122741911760, -31.23296902231887273, 14.43357722546982380 ) ) ;
#50750=CARTESIAN_POINT ( 'NONE',  ( 12.59130566666910944, -33.86016745060436506, -10.02644098062840960 ) ) ;
#50776=DIRECTION ( 'NONE',  ( 0.000000000000000000, 0.000000000000000000, -1.000000000000000000 ) ) ;
#50796=VECTOR ( 'NONE', #60040, 1000.000000000000000 ) ;
#50835=CARTESIAN_POINT ( 'NONE',  ( -15.60798173054863014, -34.17470894020248551, 7.727686298002682364 ) ) ;
#50841=CARTESIAN_POINT ( 'NONE',  ( -25.00000000000000355, -28.99999999999999645, -5.000000000000000000 ) ) ;
#50877=CARTESIAN_POINT ( 'NONE',  ( -0.9955874700083148232, -25.73414319850213161, 15.65071058219114342 ) ) ;
#50899=CARTESIAN_POINT ( 'NONE',  ( 16.71517827323052785, -28.42750353049531853, -9.642361815241612177 ) ) ;
#50900=CARTESIAN_POINT ( 'NONE',  ( -13.38666790241063964, -28.49056413965659473, 12.64716857254873617 ) ) ;
#50912=VECTOR ( 'NONE', #42060, 1000.000000000000000 ) ;
#50924=VERTEX_POINT ( 'NONE', #11063 ) ;
#50926=CARTESIAN_POINT ( 'NONE',  ( 48.22764741571069891, -0.3553121838687465228, 6.242084797467406965 ) ) ;
#50934=AXIS2_PLACEMENT_3D ( 'NONE', #38549, #13909, #8294 ) ;
#50943=CARTESIAN_POINT ( 'NONE',  ( -1.046707184715599759, -26.56309036555548886, -16.21005351936483052 ) ) ;
#50952=CARTESIAN_POINT ( 'NONE',  ( -14.83484859610010886, -34.67578963453992458, 7.338086519103280025 ) ) ;
#50971=CARTESIAN_POINT ( 'NONE',  ( -37.25000000000000711, -45.00200000000000244, 4.499999999999997335 ) ) ;
#50986=CARTESIAN_POINT ( 'NONE',  ( 50.00070814568294963, 0.0001445496031041041481, 0.7971761463862205854 ) ) ;
#50991=CARTESIAN_POINT ( 'NONE',  ( 8.434373009633013396, -31.78234095107969281, 13.63772037844789864 ) ) ;
#51012=EDGE_LOOP ( 'NONE', ( #13047, #2963, #62946, #11027 ) ) ;
#51019=CARTESIAN_POINT ( 'NONE',  ( -6.714735010819111949, -31.93429545817926751, 13.37736225704815141 ) ) ;
#51027=EDGE_LOOP ( 'NONE', ( #3020, #13231, #55599, #3387 ) ) ;
#51030=CARTESIAN_POINT ( 'NONE',  ( 14.48396081724360229, -30.02861890643185916, 3.972401191364298700 ) ) ;
#51080=CARTESIAN_POINT ( 'NONE',  ( -15.66937148611491359, -34.93011823067270427, -5.816432770871436730 ) ) ;
#51100=DIRECTION ( 'NONE',  ( 0.000000000000000000, 1.000000000000000000, 0.000000000000000000 ) ) ;
#51218=ORIENTED_EDGE ( 'NONE', *, *, #48249, .F. ) ;
#51264=CARTESIAN_POINT ( 'NONE',  ( 38.94999461337799573, -1.999059167504507739, -19.54503265464387241 ) ) ;
#51285=CARTESIAN_POINT ( 'NONE',  ( 14.27815883903287464, -30.09651741059179031, -4.806648824294282640 ) ) ;
#51294=CARTESIAN_POINT ( 'NONE',  ( -1.754394376698012570, -31.09667363889180791, 14.37851519254956756 ) ) ;
#51335=CARTESIAN_POINT ( 'NONE',  ( 13.29259107886818647, -33.36832009551446987, 10.54479676545775035 ) ) ;
#51344=ADVANCED_FACE ( 'NONE', ( #30398 ), #32981, .T. ) ;
#51364=VERTEX_POINT ( 'NONE', #23722 ) ;
#51366=CARTESIAN_POINT ( 'NONE',  ( 0.8805962972398279076, -27.81433265277922828, 12.58259205803954828 ) ) ;
#51375=ORIENTED_EDGE ( 'NONE', *, *, #32647, .T. ) ;
#51379=CARTESIAN_POINT ( 'NONE',  ( 3.616736114193262353, -30.77385512440581650, 15.02426791487729218 ) ) ;
#51393=VECTOR ( 'NONE', #6837, 1000.000000000000000 ) ;
#51455=ADVANCED_FACE ( 'NONE', ( #27954 ), #63190, .T. ) ;
#51476=DIRECTION ( 'NONE',  ( 0.000000000000000000, 0.000000000000000000, -1.000000000000000000 ) ) ;
#51540=CARTESIAN_POINT ( 'NONE',  ( -14.53304282576173279, -30.00000000000001066, 3.713578627762639250 ) ) ;
#51545=CARTESIAN_POINT ( 'NONE',  ( -28.14317553103693825, -3.466682545733132059, 23.84441711261399632 ) ) ;
#51562=VERTEX_POINT ( 'NONE', #3996 ) ;
#51574=CARTESIAN_POINT ( 'NONE',  ( 17.05919086487388725, -28.51594916623514209, -9.278936603800785221 ) ) ;
#51575=CARTESIAN_POINT ( 'NONE',  ( 13.39083528062609751, -28.49171679073737451, 12.64377518253357913 ) ) ;
#51595=CARTESIAN_POINT ( 'NONE',  ( 44.04183182023682974, -1.142706581721708803, -14.69327751537514537 ) ) ;
#51612=CARTESIAN_POINT ( 'NONE',  ( 13.91355800505865759, -33.59315906254626327, -9.938744394552985639 ) ) ;
#51655=CARTESIAN_POINT ( 'NONE',  ( 25.82596324657534126, -3.714872568654962848, 25.00000000000000711 ) ) ;
#51688=CARTESIAN_POINT ( 'NONE',  ( -0.5153900578009965594, -25.72562925869133821, 15.66323518044676000 ) ) ;
#51712=LINE ( 'NONE', #41711, #40252 ) ;
#51717=PLANE ( 'NONE',  #13966 ) ;
#51735=CARTESIAN_POINT ( 'NONE',  ( 8.006888830061562601, -32.29065697289883730, 12.88904745433947596 ) ) ;
#51742=EDGE_CURVE ( 'NONE', #16757, #8357, #16044, .T. ) ;
#51743=CARTESIAN_POINT ( 'NONE',  ( 11.27382677987933057, -33.37417574758200800, -11.09187761368031211 ) ) ;
#51813=CARTESIAN_POINT ( 'NONE',  ( -46.20808592110950741, -0.7439837506150833724, 13.26238176883679643 ) ) ;
#51868=ORIENTED_EDGE ( 'NONE', *, *, #65588, .F. ) ;
#51888=CARTESIAN_POINT ( 'NONE',  ( -3.987543989681920920, -25.89241204356462589, -15.41372194231675508 ) ) ;
#51889=CARTESIAN_POINT ( 'NONE',  ( 7.964047368509785230, -27.27321649430781392, 15.08844977892396777 ) ) ;
#51913=EDGE_LOOP ( 'NONE', ( #25324, #57412, #2441, #8807 ) ) ;
#51915=CARTESIAN_POINT ( 'NONE',  ( 40.80553070818749006, -1.699139512677865227, -18.07784515657013102 ) ) ;
#51931=CARTESIAN_POINT ( 'NONE',  ( 18.88852658721880928, -29.92669765328984255, -6.766054962673559992 ) ) ;
#51941=AXIS2_PLACEMENT_3D ( 'NONE', #12284, #2994, #42200 ) ;
#52003=CARTESIAN_POINT ( 'NONE',  ( -3.456075311296388453, -27.96820792850356341, 12.23233986317338129 ) ) ;
#52029=CARTESIAN_POINT ( 'NONE',  ( -37.25000000000000711, 5.493969937218003549E-16, -4.500000000000000888 ) ) ;
#52033=AXIS2_PLACEMENT_3D ( 'NONE', #33240, #52871, #38558 ) ;
#52039=ADVANCED_FACE ( 'NONE', ( #27699 ), #1134, .T. ) ;
#52073=DIRECTION ( 'NONE',  ( 0.2475719085175098200, -2.922992529533354589E-16, -0.9688695217174487784 ) ) ;
#52088=AXIS2_PLACEMENT_3D ( 'NONE', #11075, #30368, #20388 ) ;
#52148=CARTESIAN_POINT ( 'NONE',  ( -15.04954985558960878, -34.74586518154888637, -6.983850705393018998 ) ) ;
#52158=FACE_OUTER_BOUND ( 'NONE', #34700, .T. ) ;
#52176=VECTOR ( 'NONE', #62428, 1000.000000000000000 ) ;
#52184=CARTESIAN_POINT ( 'NONE',  ( -18.91767133624980701, -29.93867241416544189, -6.768471019338287320 ) ) ;
#52193=ORIENTED_EDGE ( 'NONE', *, *, #45729, .F. ) ;
#52212=AXIS2_PLACEMENT_3D ( 'NONE', #55785, #34507, #54808 ) ;
#52221=CARTESIAN_POINT ( 'NONE',  ( -7.856485614137358908, -26.39148214816155047, -14.61473980079826340 ) ) ;
#52243=EDGE_CURVE ( 'NONE', #52558, #9981, #26782, .T. ) ;
#52247=CARTESIAN_POINT ( 'NONE',  ( 30.43939922888039007, -3.192189569316896236, -23.38849890424057421 ) ) ;
#52253=EDGE_CURVE ( 'NONE', #44894, #64219, #58671, .T. ) ;
#52275=CARTESIAN_POINT ( 'NONE',  ( 0.8745425597524942862, -31.03649492335442872, -14.44372008463391310 ) ) ;
#52315=PLANE ( 'NONE',  #63300 ) ;
#52344=CARTESIAN_POINT ( 'NONE',  ( -5.492202615392249854, -31.64503107144835070, 13.74436444834396021 ) ) ;
#52378=VECTOR ( 'NONE', #13347, 1000.000000000000000 ) ;
#52388=CARTESIAN_POINT ( 'NONE',  ( -41.00000000000000711, -25.45369917733757603, 1.516638822270954590 ) ) ;
#52406=CARTESIAN_POINT ( 'NONE',  ( 41.00000000000000711, -45.00200000000000244, -4.500000000000000888 ) ) ;
#52461=AXIS2_PLACEMENT_3D ( 'NONE', #20578, #24573, #34845 ) ;
#52466=VERTEX_POINT ( 'NONE', #42239 ) ;
#52478=CARTESIAN_POINT ( 'NONE',  ( -42.06985574703969633, -1.486553742990790239, 18.28338660486113554 ) ) ;
#52486=CARTESIAN_POINT ( 'NONE',  ( -17.34314652423584491, -28.58740822003687754, -8.955725788651514918 ) ) ;
#52524=EDGE_CURVE ( 'NONE', #32577, #37992, #50154, .T. ) ;
#52541=AXIS2_PLACEMENT_3D ( 'NONE', #35047, #20442, #45373 ) ;
#52552=ORIENTED_EDGE ( 'NONE', *, *, #65148, .F. ) ;
#52558=VERTEX_POINT ( 'NONE', #18331 ) ;
#52564=CARTESIAN_POINT ( 'NONE',  ( 3.202861212844931416, -30.72210164159599088, -15.08749394223872642 ) ) ;
#52596=CARTESIAN_POINT ( 'NONE',  ( 8.295782569429569264, -27.33295754267981792, -14.98640435464887588 ) ) ;
#52616=EDGE_LOOP ( 'NONE', ( #9646, #61163 ) ) ;
#52624=CARTESIAN_POINT ( 'NONE',  ( 41.00000000000000711, -45.00200000000000244, 4.499999999999997335 ) ) ;
#52667=CARTESIAN_POINT ( 'NONE',  ( 9.075728589825974524, -28.84360970496452126, 9.643933591119377979 ) ) ;
#52714=CARTESIAN_POINT ( 'NONE',  ( -41.00000000000000711, -45.00200000000000244, 4.499999999999997335 ) ) ;
#52718=ORIENTED_EDGE ( 'NONE', *, *, #37311, .T. ) ;
#52722=CARTESIAN_POINT ( 'NONE',  ( -25.00000000000000355, -28.99999999999999645, 5.000000000000000888 ) ) ;
#52741=VERTEX_POINT ( 'NONE', #36554 ) ;
#52750=CARTESIAN_POINT ( 'NONE',  ( -47.72075422404362399, -0.4543357781461417333, 7.770873616088293190 ) ) ;
#52792=CARTESIAN_POINT ( 'NONE',  ( -11.75561129372955094, -29.30098385689620244, -6.671426272441853378 ) ) ;
#52816=( NAMED_UNIT ( * ) PLANE_ANGLE_UNIT ( ) SI_UNIT ( $, .RADIAN. ) );
#52871=DIRECTION ( 'NONE',  ( 0.000000000000000000, 1.000000000000000000, 0.000000000000000000 ) ) ;
#52936=ORIENTED_EDGE ( 'NONE', *, *, #33875, .T. ) ;
#52939=ADVANCED_FACE ( 'NONE', ( #59142, #8575 ), #49174, .T. ) ;
#52942=CARTESIAN_POINT ( 'NONE',  ( 14.99320290036090064, -28.92253633446381400, -11.50449902612428055 ) ) ;
#52958=LINE ( 'NONE', #62932, #22490 ) ;
#52966=EDGE_LOOP ( 'NONE', ( #12310, #2384, #61878, #42432 ) ) ;
#53014=DIRECTION ( 'NONE',  ( 1.000000000000000000, -0.000000000000000000, -0.000000000000000000 ) ) ;
#53032=DIRECTION ( 'NONE',  ( -1.000000000000000000, 0.000000000000000000, -0.000000000000000000 ) ) ;
#53057=ADVANCED_FACE ( 'NONE', ( #21168 ), #47122, .T. ) ;
#53060=CARTESIAN_POINT ( 'NONE',  ( -13.98431177871173858, -30.12623156650465006, 5.679219063900180942 ) ) ;
#53064=CARTESIAN_POINT ( 'NONE',  ( -34.90603985575356916, -2.603248520265800448, -21.87429913450488073 ) ) ;
#53083=CARTESIAN_POINT ( 'NONE',  ( 37.25000000000000711, -45.00200000000000244, 4.499999999999997335 ) ) ;
#53118=CARTESIAN_POINT ( 'NONE',  ( -12.31125281582930064, -29.30934768819284386, -5.548768499314231661 ) ) ;
#53119=ORIENTED_EDGE ( 'NONE', *, *, #52524, .F. ) ;
#53126=EDGE_LOOP ( 'NONE', ( #58356, #35730, #46149, #4414, #61852, #50278 ) ) ;
#53188=CARTESIAN_POINT ( 'NONE',  ( -19.26763262626409912, -29.00000000000001776, -5.969230316860659080 ) ) ;
#53198=CARTESIAN_POINT ( 'NONE',  ( 5.011577697822175992, -30.99110506585689251, -14.75067033891488144 ) ) ;
#53211=ORIENTED_EDGE ( 'NONE', *, *, #59439, .T. ) ;
#53237=AXIS2_PLACEMENT_3D ( 'NONE', #39061, #49412, #59690 ) ;
#53306=CIRCLE ( 'NONE', #21450, 3.999999999999999556 ) ;
#53319=CARTESIAN_POINT ( 'NONE',  ( 15.64085769076060295, -34.91570230176446898, 5.822163132929507157 ) ) ;
#53335=AXIS2_PLACEMENT_3D ( 'NONE', #30678, #61280, #47320 ) ;
#53351=ORIENTED_EDGE ( 'NONE', *, *, #58536, .T. ) ;
#53367=CARTESIAN_POINT ( 'NONE',  ( 6.824632601702067980, -31.95616727127245582, 13.35541573562488438 ) ) ;
#53398=ORIENTED_EDGE ( 'NONE', *, *, #40682, .F. ) ;
#53403=VERTEX_POINT ( 'NONE', #10703 ) ;
#53407=CARTESIAN_POINT ( 'NONE',  ( -11.13812830828974043, -32.61426855637455446, 12.21782902109530866 ) ) ;
#53412=CARTESIAN_POINT ( 'NONE',  ( -46.86486279825822265, -0.6193039491651883832, -9.927184253397708602 ) ) ;
#53455=CARTESIAN_POINT ( 'NONE',  ( -46.22120612461743860, -0.7415077656649122773, -13.24100464050678916 ) ) ;
#53460=ORIENTED_EDGE ( 'NONE', *, *, #7894, .F. ) ;
#53510=VERTEX_POINT ( 'NONE', #32942 ) ;
#53526=DIRECTION ( 'NONE',  ( 0.000000000000000000, -1.000000000000000000, 0.000000000000000000 ) ) ;
#53547=CARTESIAN_POINT ( 'NONE',  ( 1.836544102188037542, -30.58412608844215796, -15.25442441212476652 ) ) ;
#53667=EDGE_CURVE ( 'NONE', #31565, #51364, #41823, .T. ) ;
#53681=AXIS2_PLACEMENT_3D ( 'NONE', #54258, #38627, #58940 ) ;
#53694=CARTESIAN_POINT ( 'NONE',  ( 26.65194590272820108, -3.631858188236756657, -25.00000000000000711 ) ) ;
#53732=CARTESIAN_POINT ( 'NONE',  ( -10.20982488791560883, -27.71818678970603500, 14.28592212877897438 ) ) ;
#53773=ORIENTED_EDGE ( 'NONE', *, *, #54622, .F. ) ;
#53777=DIRECTION ( 'NONE',  ( 0.000000000000000000, 1.000000000000000000, 0.000000000000000000 ) ) ;
#53786=CARTESIAN_POINT ( 'NONE',  ( 3.448218607682480563, -27.97504209442909939, -12.21548802405080991 ) ) ;
#53794=ORIENTED_EDGE ( 'NONE', *, *, #54229, .F. ) ;
#53796=ORIENTED_EDGE ( 'NONE', *, *, #17577, .T. ) ;
#53814=ORIENTED_EDGE ( 'NONE', *, *, #24570, .F. ) ;
#53860=EDGE_CURVE ( 'NONE', #22226, #41515, #31566, .T. ) ;
#53904=AXIS2_PLACEMENT_3D ( 'NONE', #57583, #12004, #2037 ) ;
#53923=AXIS2_PLACEMENT_3D ( 'NONE', #4423, #34964, #49965 ) ;
#53924=FACE_OUTER_BOUND ( 'NONE', #36202, .T. ) ;
#53966=CARTESIAN_POINT ( 'NONE',  ( 15.04222346523121168, -34.74354600359600909, 6.996510958921167145 ) ) ;
#54016=AXIS2_PLACEMENT_3D ( 'NONE', #16386, #62249, #58255 ) ;
#54052=CARTESIAN_POINT ( 'NONE',  ( -7.103478058730853917, -31.43429545818073834, 14.15162322622613544 ) ) ;
#54065=EDGE_LOOP ( 'NONE', ( #15200, #13369, #30971, #16355 ) ) ;
#54071=FACE_OUTER_BOUND ( 'NONE', #28731, .T. ) ;
#54094=CARTESIAN_POINT ( 'NONE',  ( 41.00000000000000711, 1.820029539775944174E-16, -1.500000000000000222 ) ) ;
#54099=CARTESIAN_POINT ( 'NONE',  ( -9.081998980629425233, -32.61802400030150295, -12.41144404786857081 ) ) ;
#54152=DIRECTION ( 'NONE',  ( 0.2475719085175094314, 0.000000000000000000, -0.9688695217174487784 ) ) ;
#54181=CARTESIAN_POINT ( 'NONE',  ( -41.00000000000000711, -25.03188948156373783, 4.499999999999997335 ) ) ;
#54224=VERTEX_POINT ( 'NONE', #9544 ) ;
#54229=EDGE_CURVE ( 'NONE', #38939, #32577, #30180, .T. ) ;
#54233=DIRECTION ( 'NONE',  ( 0.000000000000000000, 0.000000000000000000, -1.000000000000000000 ) ) ;
#54249=AXIS2_PLACEMENT_3D ( 'NONE', #19954, #30574, #20282 ) ;
#54258=CARTESIAN_POINT ( 'NONE',  ( 0.000000000000000000, -33.00000000000000000, 0.000000000000000000 ) ) ;
#54353=ORIENTED_EDGE ( 'NONE', *, *, #35342, .F. ) ;
#54374=EDGE_CURVE ( 'NONE', #11657, #33165, #32458, .T. ) ;
#54393=CARTESIAN_POINT ( 'NONE',  ( -2.287538219536366935, -28.18941229671508708, 13.77533426008843165 ) ) ;
#54428=LINE ( 'NONE', #9485, #39610 ) ;
#54429=AXIS2_PLACEMENT_3D ( 'NONE', #44157, #39154, #19866 ) ;
#54437=DIRECTION ( 'NONE',  ( -1.000000000000000000, -0.000000000000000000, -0.000000000000000000 ) ) ;
#54443=CARTESIAN_POINT ( 'NONE',  ( 5.786001662380198418, -26.09353282112645189, -15.10027383179532023 ) ) ;
#54452=CARTESIAN_POINT ( 'NONE',  ( 25.00000000000000355, -28.99999999999999645, 5.000000000000000888 ) ) ;
#54457=FACE_OUTER_BOUND ( 'NONE', #62330, .T. ) ;
#54459=DIRECTION ( 'NONE',  ( 0.000000000000000000, 0.000000000000000000, 1.000000000000000000 ) ) ;
#54594=ORIENTED_EDGE ( 'NONE', *, *, #34360, .F. ) ;
#54596=FACE_OUTER_BOUND ( 'NONE', #19775, .T. ) ;
#54607=CARTESIAN_POINT ( 'NONE',  ( -17.14901781563217398, -29.51442629269803319, -9.398967198486927188 ) ) ;
#54622=EDGE_CURVE ( 'NONE', #50924, #48019, #31204, .T. ) ;
#54632=ORIENTED_EDGE ( 'NONE', *, *, #45930, .F. ) ;
#54642=CARTESIAN_POINT ( 'NONE',  ( -8.761386526128427832, -27.42676914488344408, -14.81571904625959135 ) ) ;
#54680=CARTESIAN_POINT ( 'NONE',  ( 36.06679944573490104, -2.440416481716450203, -22.47657575504853256 ) ) ;
#54700=AXIS2_PLACEMENT_3D ( 'NONE', #56180, #19649, #14945 ) ;
#54707=LINE ( 'NONE', #9128, #6758 ) ;
#54718=CARTESIAN_POINT ( 'NONE',  ( -1.046707184715866212, -26.56309036555506253, 16.21005351936545935 ) ) ;
#54729=CARTESIAN_POINT ( 'NONE',  ( -25.00000000000000355, -9.999999999999998224, 1.530808498934191521E-15 ) ) ;
#54754=EDGE_LOOP ( 'NONE', ( #2646, #25318, #22255, #44590, #26167, #64032 ) ) ;
#54768=CARTESIAN_POINT ( 'NONE',  ( -7.016966734453155219, -28.45964332337148406, -10.94381053768293555 ) ) ;
#54808=DIRECTION ( 'NONE',  ( 0.000000000000000000, 0.000000000000000000, 1.000000000000000000 ) ) ;
#54875=VERTEX_POINT ( 'NONE', #1044 ) ;
#54896=VERTEX_POINT ( 'NONE', #21313 ) ;
#54935=CARTESIAN_POINT ( 'NONE',  ( 3.702144525957853816, -26.71142515285320584, -15.98786919972985920 ) ) ;
#54938=ORIENTED_EDGE ( 'NONE', *, *, #54374, .F. ) ;
#54939=DIRECTION ( 'NONE',  ( 0.000000000000000000, 1.000000000000000000, 0.000000000000000000 ) ) ;
#54971=CARTESIAN_POINT ( 'NONE',  ( -41.00000000000000711, -1.694065894508600678E-18, 1.500000000000000222 ) ) ;
#54976=AXIS2_PLACEMENT_3D ( 'NONE', #14934, #60181, #4339 ) ;
#54978=CARTESIAN_POINT ( 'NONE',  ( 46.20808592110949320, -0.7439837506150870361, -13.26238176883679643 ) ) ;
#54980=CARTESIAN_POINT ( 'NONE',  ( -49.66779747649344046, -0.06758380666729577047, -4.082965791224115293 ) ) ;
#54988=VECTOR ( 'NONE', #14207, 1000.000000000000000 ) ;
#55009=CARTESIAN_POINT ( 'NONE',  ( -10.55354650058127319, -33.11426855636985778, 11.57717840647777408 ) ) ;
#55020=CARTESIAN_POINT ( 'NONE',  ( 14.79723931605636444, -33.90329588773487757, 8.884483617263549959 ) ) ;
#55033=EDGE_CURVE ( 'NONE', #27125, #52558, #42918, .T. ) ;
#55054=DIRECTION ( 'NONE',  ( -0.000000000000000000, -0.000000000000000000, -1.000000000000000000 ) ) ;
#55071=CARTESIAN_POINT ( 'NONE',  ( -5.492202615392249854, -31.64503107144835070, -13.74436444834396021 ) ) ;
#55155=CARTESIAN_POINT ( 'NONE',  ( -14.82142464308439322, -33.91165328791086608, 8.853132628085452538 ) ) ;
#55185=DIRECTION ( 'NONE',  ( 0.000000000000000000, 1.000000000000000000, 0.000000000000000000 ) ) ;
#55197=CARTESIAN_POINT ( 'NONE',  ( 3.474069148988125466, -25.85800187936594341, 15.46552914816621005 ) ) ;
#55217=FACE_OUTER_BOUND ( 'NONE', #39895, .T. ) ;
#55222=CARTESIAN_POINT ( 'NONE',  ( -19.56743653832047514, -30.00000000000000000, 5.000000000000000888 ) ) ;
#55232=CARTESIAN_POINT ( 'NONE',  ( -15.75855542457931335, -29.13485235466247403, -10.82860303369087873 ) ) ;
#55262=CARTESIAN_POINT ( 'NONE',  ( -3.650755842799267459, -28.29207189712390402, -13.56609188631114193 ) ) ;
#55264=CARTESIAN_POINT ( 'NONE',  ( 40.99999999999999289, -25.49182303066451993, -1.512869109757712716 ) ) ;
#55295=ORIENTED_EDGE ( 'NONE', *, *, #25301, .T. ) ;
#55306=CARTESIAN_POINT ( 'NONE',  ( 46.64267184946613298, -0.6617291737840894639, 12.54075111122643804 ) ) ;
#55335=ORIENTED_EDGE ( 'NONE', *, *, #64334, .F. ) ;
#55339=CARTESIAN_POINT ( 'NONE',  ( -41.00000000000000711, -25.03188948156373783, 4.499999999999997335 ) ) ;
#55343=CARTESIAN_POINT ( 'NONE',  ( -18.91767133624980701, -28.94173879345719058, 6.680047468371234309 ) ) ;
#55355=CARTESIAN_POINT ( 'NONE',  ( 11.12775972613914099, -27.93149659178545008, 13.86083901436676591 ) ) ;
#55360=ORIENTED_EDGE ( 'NONE', *, *, #48366, .F. ) ;
#55404=CARTESIAN_POINT ( 'NONE',  ( 13.74768401152558894, -27.65692779101644305, -12.04119239038937117 ) ) ;
#55417=ORIENTED_EDGE ( 'NONE', *, *, #31723, .T. ) ;
#55438=FACE_OUTER_BOUND ( 'NONE', #31894, .T. ) ;
#55441=EDGE_LOOP ( 'NONE', ( #12552, #64590, #41804, #11597 ) ) ;
#55492=DIRECTION ( 'NONE',  ( -1.000000000000000000, 0.000000000000000000, 0.000000000000000000 ) ) ;
#55497=ORIENTED_EDGE ( 'NONE', *, *, #57273, .T. ) ;
#55509=EDGE_CURVE ( 'NONE', #49767, #9981, #44181, .T. ) ;
#55536=CARTESIAN_POINT ( 'NONE',  ( 4.953976645022758696, -25.99587143922707000, 15.25378271594937019 ) ) ;
#55564=CARTESIAN_POINT ( 'NONE',  ( -16.81808179455697783, -29.42526233323303586, 9.774508714121763475 ) ) ;
#55576=CARTESIAN_POINT ( 'NONE',  ( -14.60253471108646117, -28.81751583403978501, -11.78204505887442011 ) ) ;
#55599=ORIENTED_EDGE ( 'NONE', *, *, #51742, .F. ) ;
#55610=CARTESIAN_POINT ( 'NONE',  ( 3.168054457075692554, -30.71813892570141036, -15.09231838820015170 ) ) ;
#55620=CARTESIAN_POINT ( 'NONE',  ( -8.419536088379066641, -32.40770164630938410, 12.72556558505709212 ) ) ;
#55633=CARTESIAN_POINT ( 'NONE',  ( -25.00000000000000355, -28.99999999999999645, -5.000000000000000888 ) ) ;
#55657=EDGE_LOOP ( 'NONE', ( #65346, #6954 ) ) ;
#55659=CARTESIAN_POINT ( 'NONE',  ( 15.08189101924520870, -34.00125857029218679, 8.507794521696036227 ) ) ;
#55683=CARTESIAN_POINT ( 'NONE',  ( -11.18139917412363182, -29.23077454460525360, 7.530122743832658117 ) ) ;
#55694=CARTESIAN_POINT ( 'NONE',  ( 15.59065549519832494, -34.16917994668085612, 7.755393724195712934 ) ) ;
#55743=CARTESIAN_POINT ( 'NONE',  ( 8.754896909465220034, -28.78086681028207749, -9.883947858767701433 ) ) ;
#55744=ORIENTED_EDGE ( 'NONE', *, *, #59149, .T. ) ;
#55766=B_SPLINE_CURVE_WITH_KNOTS ( 'NONE', 3,
 ( #30952, #61874, #61222, #52247, #15647, #56221, #35614, #10665, #391, #51264, #31602, #51915, #41914, #6356, #51595, #10338, #26624, #5715, #40607, #6688, #25986, #55907, #6044, #21658, #46271, #62198, #30614, #41250, #26301, #61532, #47261, #46918, #1702, #50926, #46581, #1036, #16333, #36607, #15974, #36922, #21306, #41584, #16651, #5371, #48258, #17314, #38225, #33253, #2014, #48567, #32903, #63827, #2361, #47567 ),
 .UNSPECIFIED., .F., .F.,
 ( 4, 2, 2, 2, 2, 2, 2, 2, 2, 2, 2, 2, 2, 2, 2, 2, 2, 2, 2, 2, 2, 2, 2, 2, 2, 2, 4 ),
 ( 0.000000000000000000, 0.004712545709777831403, 0.007068818564666746670, 0.009425091419555662806, 0.01413763712933349681, 0.01649390998422241295, 0.01885018283911132908, 0.02356272854888913360, 0.02591900140377803932, 0.02827527425866694158, 0.03063154711355584384, 0.03180968354100029150, 0.03298781996844474262, 0.03770036567822253326, 0.04005663853311142858, 0.04123477496055587971, 0.04241291138800033084, 0.04712545709777812841, 0.04948172995266704455, 0.05183800280755595374, 0.05655054851733376520, 0.06126309422711157665, 0.06361936708200048585, 0.06597563993688938810, 0.07068818564666720650, 0.07304445850155609488, 0.07540073135644499713 ),
 .UNSPECIFIED. ) ;
#55785=CARTESIAN_POINT ( 'NONE',  ( 0.000000000000000000, -33.00000000000000000, 0.000000000000000000 ) ) ;
#55799=DIRECTION ( 'NONE',  ( 0.9688695217174486674, 1.734723475976807292E-15, -0.2475719085175099865 ) ) ;
#55818=B_SPLINE_CURVE_WITH_KNOTS ( 'NONE', 3,
 ( #8076, #18391, #11804, #33660, #8726, #24024 ),
 .UNSPECIFIED., .F., .F.,
 ( 4, 2, 4 ),
 ( 0.006113759649309998857, 0.008271820019582997591, 0.01042988038985599719 ),
 .UNSPECIFIED. ) ;
#55864=CARTESIAN_POINT ( 'NONE',  ( 9.722110222095130538, -26.73349363795547973, 14.00621188957225449 ) ) ;
#55878=DIRECTION ( 'NONE',  ( 0.000000000000000000, 0.000000000000000000, 1.000000000000000000 ) ) ;
#55886=CARTESIAN_POINT ( 'NONE',  ( -2.024814117303733063, -26.59886070765379529, 16.15701038285739344 ) ) ;
#55907=CARTESIAN_POINT ( 'NONE',  ( 48.06591103469481396, -0.3868811097602622984, -6.642178517338836130 ) ) ;
#55924=CARTESIAN_POINT ( 'NONE',  ( -5.813762929211843122, -31.14503107144930638, -14.54886001617044222 ) ) ;
#55935=CARTESIAN_POINT ( 'NONE',  ( -25.00000000000000355, -3.797884998337192286, 23.99999999999999289 ) ) ;
#55960=DIRECTION ( 'NONE',  ( -1.000000000000000000, -0.000000000000000000, -0.000000000000000000 ) ) ;
#55975=EDGE_CURVE ( 'NONE', #16757, #65704, #28454, .T. ) ;
#55995=CARTESIAN_POINT ( 'NONE',  ( -19.30028080049353179, -29.00000000000000000, 5.863682654924961213 ) ) ;
#56006=CARTESIAN_POINT ( 'NONE',  ( 13.91355800505865759, -33.59315906254626327, 9.938744394552985639 ) ) ;
#56048=CARTESIAN_POINT ( 'NONE',  ( 15.96609733983705226, -34.98269025770574103, -4.990963945245213473 ) ) ;
#56177=CARTESIAN_POINT ( 'NONE',  ( 10.63650944684269994, -26.92414420718871426, 13.64813004266018481 ) ) ;
#56180=CARTESIAN_POINT ( 'NONE',  ( 22.00000000000000711, -20.00000000000000000, 2.449293598294706907E-15 ) ) ;
#56196=CARTESIAN_POINT ( 'NONE',  ( -38.56928140186734311, -26.58605982982061633, -4.500000000000001776 ) ) ;
#56197=( LENGTH_UNIT ( ) NAMED_UNIT ( * ) SI_UNIT ( .MILLI., .METRE. ) );
#56221=CARTESIAN_POINT ( 'NONE',  ( 32.70177428389710172, -2.904144763113409411, -22.74422317523287163 ) ) ;
#56240=CARTESIAN_POINT ( 'NONE',  ( 11.32820571420733735, -29.68697874620919563, -9.642237626533519901 ) ) ;
#56250=CARTESIAN_POINT ( 'NONE',  ( -5.596759081073452435, -31.66776075797034196, 13.71641508080542771 ) ) ;
#56285=CARTESIAN_POINT ( 'NONE',  ( 48.71973356879950501, -0.2586908456632806552, 8.066649094095312833 ) ) ;
#56318=DIRECTION ( 'NONE',  ( 0.000000000000000000, 0.000000000000000000, -1.000000000000000000 ) ) ;
#56319=CARTESIAN_POINT ( 'NONE',  ( -13.50035326695106797, -34.20038524408859359, 9.091202907900893138 ) ) ;
#56330=CARTESIAN_POINT ( 'NONE',  ( 5.268658153349320195, -26.87458176590442704, 15.73590792199922461 ) ) ;
#56370=ORIENTED_EDGE ( 'NONE', *, *, #64874, .T. ) ;
#56373=CARTESIAN_POINT ( 'NONE',  ( 14.06742311317152172, -34.40796758970507341, 8.422011900743699542 ) ) ;
#56381=CIRCLE ( 'NONE', #3299, 5.000000000000001776 ) ;
#56481=PLANE ( 'NONE',  #25493 ) ;
#56486=CARTESIAN_POINT ( 'NONE',  ( -25.00000000000000355, -3.797884998337192286, 24.99999999999999289 ) ) ;
#56502=CARTESIAN_POINT ( 'NONE',  ( -14.80332308495294136, -33.90539544390878035, 8.876538241603904922 ) ) ;
#56507=CARTESIAN_POINT ( 'NONE',  ( -33.44920912455759066, -2.804301875032225499, 22.47723755754419628 ) ) ;
#56525=ORIENTED_EDGE ( 'NONE', *, *, #18267, .F. ) ;
#56541=AXIS2_PLACEMENT_3D ( 'NONE', #43367, #53032, #7467 ) ;
#56556=CARTESIAN_POINT ( 'NONE',  ( 37.25000000000000711, -20.00000000000000000, 1.500000000000002887 ) ) ;
#56569=DIRECTION ( 'NONE',  ( 0.000000000000000000, 0.000000000000000000, -1.000000000000000000 ) ) ;
#56589=CARTESIAN_POINT ( 'NONE',  ( 16.25880638383053167, -34.36679772354877116, -6.546306705357506139 ) ) ;
#56641=CARTESIAN_POINT ( 'NONE',  ( 47.41189015808931373, -0.5144011408980397881, -11.10762064040663510 ) ) ;
#56678=CARTESIAN_POINT ( 'NONE',  ( 11.27382677987933057, -33.37417574758200800, 11.09187761368031211 ) ) ;
#56691=DIRECTION ( 'NONE',  ( 0.000000000000000000, 0.000000000000000000, 1.000000000000000000 ) ) ;
#56737=CARTESIAN_POINT ( 'NONE',  ( 8.395146353829712638, -32.40713589851873166, 12.72020452407952540 ) ) ;
#56744=CARTESIAN_POINT ( 'NONE',  ( 9.989421171649008002, -29.02163280020721103, -8.890648868200056398 ) ) ;
#56809=EDGE_LOOP ( 'NONE', ( #54594, #58487, #29047, #63196 ) ) ;
#56852=CARTESIAN_POINT ( 'NONE',  ( 41.00000000000000711, -25.18551001833412784, 3.766049837354531693 ) ) ;
#56878=( GEOMETRIC_REPRESENTATION_CONTEXT ( 3 ) GLOBAL_UNCERTAINTY_ASSIGNED_CONTEXT ( ( #64196 ) ) GLOBAL_UNIT_ASSIGNED_CONTEXT ( ( #50125, #59436, #33824 ) ) REPRESENTATION_CONTEXT ( 'NONE', 'WORKASPACE' ) );
#56888=CARTESIAN_POINT ( 'NONE',  ( 6.904443316226203109, -26.24011843744382233, -14.86481251185162655 ) ) ;
#56889=CARTESIAN_POINT ( 'NONE',  ( 17.13446681924521187, -29.51054447109572365, 9.416006455614706283 ) ) ;
#56929=CARTESIAN_POINT ( 'NONE',  ( 17.33919137821675349, -29.56463768738087694, -9.168593624349773208 ) ) ;
#56931=VERTEX_POINT ( 'NONE', #3650 ) ;
#56937=CARTESIAN_POINT ( 'NONE',  ( -13.24204686117196950, -34.10419274375099974, 9.367294588221389162 ) ) ;
#56985=ORIENTED_EDGE ( 'NONE', *, *, #32919, .T. ) ;
#56988=ADVANCED_FACE ( 'NONE', ( #44174 ), #62545, .F. ) ;
#56997=CARTESIAN_POINT ( 'NONE',  ( 5.786001662380198418, -26.09353282112645189, 15.10027383179532023 ) ) ;
#57070=CARTESIAN_POINT ( 'NONE',  ( -22.00000000000000711, -20.00000000000000000, 2.449293598294706907E-15 ) ) ;
#57101=CIRCLE ( 'NONE', #7141, 20.19615242270663558 ) ;
#57129=CARTESIAN_POINT ( 'NONE',  ( -39.53125591517013504, -1.906753238347176582, 20.35939770057402498 ) ) ;
#57135=CARTESIAN_POINT ( 'NONE',  ( -19.56743653832047158, -29.00000000000000000, -5.000000000000000888 ) ) ;
#57203=CARTESIAN_POINT ( 'NONE',  ( 19.41740522748896680, -28.99999999999999645, -5.485033347092790557 ) ) ;
#57219=VECTOR ( 'NONE', #32991, 1000.000000000000000 ) ;
#57225=FACE_OUTER_BOUND ( 'NONE', #64109, .T. ) ;
#57238=CARTESIAN_POINT ( 'NONE',  ( 25.00000000000000711, -9.999999999999998224, -24.00000000000000000 ) ) ;
#57273=EDGE_CURVE ( 'NONE', #61621, #65150, #19745, .T. ) ;
#57274=VERTEX_POINT ( 'NONE', #34364 ) ;
#57280=AXIS2_PLACEMENT_3D ( 'NONE', #17982, #17665, #32588 ) ;
#57316=CARTESIAN_POINT ( 'NONE',  ( -2.136460567204509164, -31.12783502484143128, 14.34456412933875846 ) ) ;
#57345=AXIS2_PLACEMENT_3D ( 'NONE', #31660, #21030, #46642 ) ;
#57359=DIRECTION ( 'NONE',  ( -1.000000000000000000, 0.000000000000000000, 0.000000000000000000 ) ) ;
#57402=EDGE_CURVE ( 'NONE', #30420, #11603, #9516, .T. ) ;
#57412=ORIENTED_EDGE ( 'NONE', *, *, #39849, .T. ) ;
#57424=ORIENTED_EDGE ( 'NONE', *, *, #50453, .F. ) ;
#57439=EDGE_LOOP ( 'NONE', ( #39080, #42065 ) ) ;
#57462=CARTESIAN_POINT ( 'NONE',  ( -18.19295774167957447, -28.79006254106626272, -7.843687167517533254 ) ) ;
#57497=FACE_OUTER_BOUND ( 'NONE', #45587, .T. ) ;
#57514=DIRECTION ( 'NONE',  ( 0.000000000000000000, 0.000000000000000000, 1.000000000000000000 ) ) ;
#57523=ADVANCED_FACE ( 'NONE', ( #17699 ), #47309, .F. ) ;
#57583=CARTESIAN_POINT ( 'NONE',  ( 0.000000000000000000, -33.00000000000000000, 0.000000000000000000 ) ) ;
#57600=ADVANCED_FACE ( 'NONE', ( #54596 ), #18696, .F. ) ;
#57659=CARTESIAN_POINT ( 'NONE',  ( 8.309432179406254448, -32.38110954670829500, 12.75850010368669629 ) ) ;
#57676=DIRECTION ( 'NONE',  ( 0.000000000000000000, -1.000000000000000000, 0.000000000000000000 ) ) ;
#57691=AXIS2_PLACEMENT_3D ( 'NONE', #8360, #63228, #59899 ) ;
#57714=CARTESIAN_POINT ( 'NONE',  ( 37.00000000000000711, -45.00200000000000244, -4.500000000000000888 ) ) ;
#57736=EDGE_CURVE ( 'NONE', #54896, #33819, #59329, .T. ) ;
#57749=EDGE_CURVE ( 'NONE', #43541, #25095, #24674, .T. ) ;
#57750=CARTESIAN_POINT ( 'NONE',  ( -43.07244751019905493, -1.315220855092201324, -15.87097690372580061 ) ) ;
#57829=EDGE_CURVE ( 'NONE', #53403, #31959, #31271, .T. ) ;
#57833=CARTESIAN_POINT ( 'NONE',  ( -13.91099446267240225, -33.59051099066058299, -9.908177736481542652 ) ) ;
#57859=LINE ( 'NONE', #12932, #36331 ) ;
#57881=EDGE_LOOP ( 'NONE', ( #47178, #26956 ) ) ;
#57969=EDGE_CURVE ( 'NONE', #62996, #41515, #45501, .T. ) ;
#57983=CARTESIAN_POINT ( 'NONE',  ( -4.254071763051084254, -31.39562805149797597, 14.04524613008041811 ) ) ;
#57995=EDGE_LOOP ( 'NONE', ( #64724, #44803, #17265, #23110 ) ) ;
#58064=CARTESIAN_POINT ( 'NONE',  ( -13.86128969992323334, -30.12619713135721611, 5.984278774111453814 ) ) ;
#58109=CARTESIAN_POINT ( 'NONE',  ( -43.79915462856099850, -1.187172983101275836, 16.56021102286109326 ) ) ;
#58146=CARTESIAN_POINT ( 'NONE',  ( -13.86128969992320847, -30.12619713135532251, -5.984278774113396260 ) ) ;
#58189=VECTOR ( 'NONE', #17518, 1000.000000000000000 ) ;
#58214=ORIENTED_EDGE ( 'NONE', *, *, #49745, .T. ) ;
#58255=DIRECTION ( 'NONE',  ( -1.000000000000000000, 0.000000000000000000, 0.000000000000000000 ) ) ;
#58265=CARTESIAN_POINT ( 'NONE',  ( 12.54355452190762144, -28.27128177340750526, -13.14909765253698559 ) ) ;
#58286=UNCERTAINTY_MEASURE_WITH_UNIT (LENGTH_MEASURE( 1.000000000000000082E-05 ), #42479, 'distance_accuracy_value', 'NONE');
#58302=CARTESIAN_POINT ( 'NONE',  ( 11.77510182854060439, -29.30972061338670187, 6.669332763617590309 ) ) ;
#58324=B_SPLINE_CURVE_WITH_KNOTS ( 'NONE', 3,
 ( #31742, #31436, #10165, #6180, #30444, #25799, #16482, #46092, #56373, #4872, #21116, #850, #25138, #41392, #36423, #56737, #51735, #53367, #32402, #33060, #37062, #27749, #7815, #62652 ),
 .UNSPECIFIED., .F., .F.,
 ( 4, 2, 2, 2, 2, 2, 2, 2, 2, 2, 2, 4 ),
 ( 0.000000000000000000, 0.001335873637788843014, 0.002671747275577686029, 0.004007620913366529043, 0.005343494551155374660, 0.008015241826733065025, 0.01068698910231075626, 0.01202286274009960361, 0.01335873637788844923, 0.01603048365346615087, 0.01870223092904384904, 0.02137397820462155415 ),
 .UNSPECIFIED. ) ;
#58356=ORIENTED_EDGE ( 'NONE', *, *, #31015, .T. ) ;
#58387=CARTESIAN_POINT ( 'NONE',  ( -13.03183108261633549, -30.03462372422968940, 7.545134388564851413 ) ) ;
#58392=DIRECTION ( 'NONE',  ( 0.000000000000000000, 0.000000000000000000, 1.000000000000000000 ) ) ;
#58436=CARTESIAN_POINT ( 'NONE',  ( -40.19089168456216754, -1.800105668799816039, 19.87241647152734458 ) ) ;
#58444=CARTESIAN_POINT ( 'NONE',  ( -11.25859294448574666, -33.36858074101470351, -11.10377723166772768 ) ) ;
#58453=ORIENTED_EDGE ( 'NONE', *, *, #43993, .T. ) ;
#58487=ORIENTED_EDGE ( 'NONE', *, *, #43169, .T. ) ;
#58494=EDGE_CURVE ( 'NONE', #8357, #62996, #14728, .T. ) ;
#58527=DIRECTION ( 'NONE',  ( -1.000000000000000000, 0.000000000000000000, 0.000000000000000000 ) ) ;
#58536=EDGE_CURVE ( 'NONE', #32724, #54875, #49894, .T. ) ;
#58541=ORIENTED_EDGE ( 'NONE', *, *, #20166, .F. ) ;
#58641=ORIENTED_EDGE ( 'NONE', *, *, #18269, .F. ) ;
#58649=CARTESIAN_POINT ( 'NONE',  ( 18.88852658721791045, -28.93036277062534012, 6.677752214540050524 ) ) ;
#58655=VERTEX_POINT ( 'NONE', #9567 ) ;
#58671=CIRCLE ( 'NONE', #45880, 250.0000000000000000 ) ;
#58719=ORIENTED_EDGE ( 'NONE', *, *, #16087, .T. ) ;
#58727=DIRECTION ( 'NONE',  ( -1.000000000000000000, 0.000000000000000000, 0.000000000000000000 ) ) ;
#58737=CARTESIAN_POINT ( 'NONE',  ( -0.4456450841876061775, -28.11949765475245400, 13.91469577634640231 ) ) ;
#58743=PLANE ( 'NONE',  #16094 ) ;
#58756=CIRCLE ( 'NONE', #10983, 1.500000000000000444 ) ;
#58757=CARTESIAN_POINT ( 'NONE',  ( -37.25000000000002132, -27.32965888902625196, 3.759436751556509915 ) ) ;
#58768=CARTESIAN_POINT ( 'NONE',  ( -22.00000000000000711, -20.00000000000000000, -1.499999999999998002 ) ) ;
#58783=FACE_OUTER_BOUND ( 'NONE', #62726, .T. ) ;
#58793=CARTESIAN_POINT ( 'NONE',  ( -3.416103270178013407, -31.26314776370590209, -14.19449313401761081 ) ) ;
#58803=DIRECTION ( 'NONE',  ( -1.000000000000000000, 0.000000000000000000, 0.000000000000000000 ) ) ;
#58839=DIRECTION ( 'NONE',  ( -0.9688695217174484453, 0.000000000000000000, 0.2475719085175105139 ) ) ;
#58940=DIRECTION ( 'NONE',  ( 0.000000000000000000, 0.000000000000000000, 1.000000000000000000 ) ) ;
#59007=FACE_OUTER_BOUND ( 'NONE', #22984, .T. ) ;
#59020=ORIENTED_EDGE ( 'NONE', *, *, #22438, .F. ) ;
#59041=EDGE_CURVE ( 'NONE', #2269, #34549, #11660, .T. ) ;
#59057=CARTESIAN_POINT ( 'NONE',  ( -13.72965000697191584, -28.58137455677819361, 12.42479717943507822 ) ) ;
#59077=CARTESIAN_POINT ( 'NONE',  ( -37.25000000000000711, -27.21021009056489248, -4.500000000000000888 ) ) ;
#59108=CARTESIAN_POINT ( 'NONE',  ( -4.254071763051084254, -31.39562805149797597, -14.04524613008041811 ) ) ;
#59142=FACE_BOUND ( 'NONE', #49732, .T. ) ;
#59149=EDGE_CURVE ( 'NONE', #9981, #14466, #5489, .T. ) ;
#59164=ADVANCED_FACE ( 'NONE', ( #14979 ), #34612, .F. ) ;
#59184=ORIENTED_EDGE ( 'NONE', *, *, #8057, .F. ) ;
#59186=CARTESIAN_POINT ( 'NONE',  ( -0.4601472316358399817, -30.53649492335484439, 15.30974548841791183 ) ) ;
#59222=CARTESIAN_POINT ( 'NONE',  ( -11.92921645562753064, -32.88698380610600935, -11.67323352594349650 ) ) ;
#59283=CARTESIAN_POINT ( 'NONE',  ( 12.59130566666910944, -33.86016745060436506, 10.02644098062840960 ) ) ;
#59329=CIRCLE ( 'NONE', #7299, 16.73205080756888563 ) ;
#59363=CARTESIAN_POINT ( 'NONE',  ( -9.369086346424605694, -29.24458096581515321, 11.21746676166726786 ) ) ;
#59410=CARTESIAN_POINT ( 'NONE',  ( 3.024435290549866817, -27.93754772256033903, -12.30283293119135202 ) ) ;
#59436=( NAMED_UNIT ( * ) PLANE_ANGLE_UNIT ( ) SI_UNIT ( $, .RADIAN. ) );
#59439=EDGE_CURVE ( 'NONE', #14466, #64767, #22288, .T. ) ;
#59505=AXIS2_PLACEMENT_3D ( 'NONE', #249, #4587, #24857 ) ;
#59516=DIRECTION ( 'NONE',  ( 0.000000000000000000, 0.000000000000000000, -1.000000000000000000 ) ) ;
#59540=CARTESIAN_POINT ( 'NONE',  ( -3.683412895348672667, -30.77133338175875465, -15.02788192792846189 ) ) ;
#59542=DIRECTION ( 'NONE',  ( -1.000000000000000000, -0.000000000000000000, -0.000000000000000000 ) ) ;
#59550=VERTEX_POINT ( 'NONE', #54181 ) ;
#59553=AXIS2_PLACEMENT_3D ( 'NONE', #63212, #59542, #54233 ) ;
#59558=CARTESIAN_POINT ( 'NONE',  ( -25.00000000000000355, -30.00000000000000000, 1.530808498934191521E-15 ) ) ;
#59574=CARTESIAN_POINT ( 'NONE',  ( -25.00000000000000355, -30.00000000000000000, 1.530808498934191521E-15 ) ) ;
#59575=CIRCLE ( 'NONE', #9667, 25.00000000000000000 ) ;
#59595=EDGE_CURVE ( 'NONE', #52466, #54224, #46793, .T. ) ;
#59608=CARTESIAN_POINT ( 'NONE',  ( 0.9290584433855355595, -28.11997881881914196, -13.91374373156083166 ) ) ;
#59690=DIRECTION ( 'NONE',  ( 0.000000000000000000, 0.000000000000000000, 1.000000000000000000 ) ) ;
#59698=CARTESIAN_POINT ( 'NONE',  ( -7.454036404615679956, -28.85515183291106212, 12.27947133142187219 ) ) ;
#59745=CARTESIAN_POINT ( 'NONE',  ( -10.20982488791560883, -26.83227745022078992, -13.82162602233992565 ) ) ;
#59827=DIRECTION ( 'NONE',  ( 0.000000000000000000, -1.000000000000000000, 0.000000000000000000 ) ) ;
#59850=DIRECTION ( 'NONE',  ( 1.000000000000000000, -0.000000000000000000, -0.000000000000000000 ) ) ;
#59859=FACE_OUTER_BOUND ( 'NONE', #51012, .T. ) ;
#59875=ORIENTED_EDGE ( 'NONE', *, *, #29951, .F. ) ;
#59899=DIRECTION ( 'NONE',  ( 0.000000000000000000, 0.000000000000000000, 1.000000000000000000 ) ) ;
#59946=CARTESIAN_POINT ( 'NONE',  ( -2.264138978095799448, -30.62783502483855358, -15.20150737401304575 ) ) ;
#59966=EDGE_LOOP ( 'NONE', ( #22520, #59020 ) ) ;
#59968=ORIENTED_EDGE ( 'NONE', *, *, #34360, .T. ) ;
#59983=CARTESIAN_POINT ( 'NONE',  ( 0.000000000000000000, -35.00000000000000000, 0.000000000000000000 ) ) ;
#59987=CARTESIAN_POINT ( 'NONE',  ( 42.06985574703970343, -1.486553742990792681, -18.28338660486113909 ) ) ;
#60016=CARTESIAN_POINT ( 'NONE',  ( -11.38801898431830040, -29.26006678106075753, 7.242958320504926384 ) ) ;
#60027=CARTESIAN_POINT ( 'NONE',  ( 16.93571557946443562, -34.49999999976442666, 4.804977935187394245 ) ) ;
#60040=DIRECTION ( 'NONE',  ( 0.000000000000000000, 1.000000000000000000, 0.000000000000000000 ) ) ;
#60054=DIRECTION ( 'NONE',  ( 1.000000000000000000, -0.000000000000000000, -0.000000000000000000 ) ) ;
#60067=CARTESIAN_POINT ( 'NONE',  ( -5.596759081085386889, -31.66776075797297096, -13.71641508080218230 ) ) ;
#60072=CARTESIAN_POINT ( 'NONE',  ( 0.8805962972398277966, -27.81433265277922828, -12.58259205804047021 ) ) ;
#60142=DIRECTION ( 'NONE',  ( 0.000000000000000000, 0.000000000000000000, -1.000000000000000000 ) ) ;
#60181=DIRECTION ( 'NONE',  ( 1.000000000000000000, 0.000000000000000000, -0.000000000000000000 ) ) ;
#60222=CARTESIAN_POINT ( 'NONE',  ( -16.12286248669608213, -29.23548504417002647, -10.48934106169928704 ) ) ;
#60247=ORIENTED_EDGE ( 'NONE', *, *, #28382, .T. ) ;
#60249=CARTESIAN_POINT ( 'NONE',  ( -0.4456450841876022362, -28.11949765475245400, -13.91469577634640231 ) ) ;
#60295=CARTESIAN_POINT ( 'NONE',  ( 46.63605190621407104, -0.6629852496305267406, -12.55202432522571421 ) ) ;
#60298=CARTESIAN_POINT ( 'NONE',  ( -43.82484328533829654, -1.182663722159860376, -16.53294353590084143 ) ) ;
#60324=CARTESIAN_POINT ( 'NONE',  ( -12.85491158824215141, -29.00000000000000711, 3.284771503683518556 ) ) ;
#60334=DIRECTION ( 'NONE',  ( 0.000000000000000000, 0.000000000000000000, 1.000000000000000000 ) ) ;
#60335=CARTESIAN_POINT ( 'NONE',  ( 13.40144019692491995, -30.08877117594913742, 6.927253557473016521 ) ) ;
#60336=VECTOR ( 'NONE', #38522, 1000.000000000000000 ) ;
#60363=AXIS2_PLACEMENT_3D ( 'NONE', #63468, #12945, #8943 ) ;
#60368=DIRECTION ( 'NONE',  ( 0.000000000000000000, 1.000000000000000000, -0.000000000000000000 ) ) ;
#60377=CARTESIAN_POINT ( 'NONE',  ( -2.195494320951781653, -31.13300424730296001, -14.33890400575618074 ) ) ;
#60379=TOROIDAL_SURFACE ( 'NONE', #15795, 20.19615242270663558, 4.000000000000000000 ) ;
#60385=CARTESIAN_POINT ( 'NONE',  ( 11.12775972613914099, -27.03492176219597454, -13.41779706364883396 ) ) ;
#60409=ADVANCED_FACE ( 'NONE', ( #65296 ), #47891, .T. ) ;
#60472=DIRECTION ( 'NONE',  ( 0.000000000000000000, 1.000000000000000000, 0.000000000000000000 ) ) ;
#60514=CYLINDRICAL_SURFACE ( 'NONE', #54700, 1.500000000000000444 ) ;
#60543=CARTESIAN_POINT ( 'NONE',  ( -19.56743653832046803, -30.00000000000000000, -5.000000000000000888 ) ) ;
#60576=CARTESIAN_POINT ( 'NONE',  ( -7.529925403076002333, -31.54078451673387917, -13.99923386364710609 ) ) ;
#60626=CARTESIAN_POINT ( 'NONE',  ( -37.50900221036945226, -2.222235401316478232, -21.66089349574501455 ) ) ;
#60659=CARTESIAN_POINT ( 'NONE',  ( -11.91618201078742523, -29.31229682091932176, 6.386286639733019577 ) ) ;
#60673=CARTESIAN_POINT ( 'NONE',  ( 11.15801620995519805, -32.62087690404786144, 12.20531625113500596 ) ) ;
#60688=TOROIDAL_SURFACE ( 'NONE', #52212, 20.19615242270663558, 3.000000000000000000 ) ;
#60724=CARTESIAN_POINT ( 'NONE',  ( 17.91771366450749525, -28.72671386922736758, -8.232269603669239544 ) ) ;
#60754=CARTESIAN_POINT ( 'NONE',  ( 41.00000000000000711, -1.694065894508600678E-18, 0.000000000000000000 ) ) ;
#60811=EDGE_CURVE ( 'NONE', #9981, #8357, #3255, .T. ) ;
#60815=EDGE_LOOP ( 'NONE', ( #62271, #40286, #30015, #637 ) ) ;
#60852=CARTESIAN_POINT ( 'NONE',  ( -14.88966238093840921, -27.95127710492162265, 11.23339344092909897 ) ) ;
#60876=CARTESIAN_POINT ( 'NONE',  ( -7.961359079021516294, -27.27258404549932536, 15.08967732372090964 ) ) ;
#60899=CARTESIAN_POINT ( 'NONE',  ( -41.00000000000000711, 5.493969937218003549E-16, -4.500000000000000888 ) ) ;
#60920=CARTESIAN_POINT ( 'NONE',  ( 4.972137933589803716, -28.45452681573965137, -13.21946257706011174 ) ) ;
#60939=VERTEX_POINT ( 'NONE', #54452 ) ;
#60967=CARTESIAN_POINT ( 'NONE',  ( 41.49302228377221979, -1.586477970524126313, 18.85982933713411569 ) ) ;
#60996=PLANE ( 'NONE',  #4552 ) ;
#60997=CARTESIAN_POINT ( 'NONE',  ( -6.641947195041168150, -28.39580239767160919, 11.12859478088952336 ) ) ;
#61007=CARTESIAN_POINT ( 'NONE',  ( 19.27363075669222425, -29.98494805059729984, 5.891112176854364613 ) ) ;
#61088=EDGE_CURVE ( 'NONE', #43036, #12741, #53306, .T. ) ;
#61163=ORIENTED_EDGE ( 'NONE', *, *, #25231, .F. ) ;
#61171=ORIENTED_EDGE ( 'NONE', *, *, #57402, .T. ) ;
#61222=CARTESIAN_POINT ( 'NONE',  ( 28.14317553103694181, -3.466682545733132503, -23.84441711261399988 ) ) ;
#61236=CARTESIAN_POINT ( 'NONE',  ( 15.07617326819549142, -33.99933334076585112, -8.515830899730527648 ) ) ;
#61280=DIRECTION ( 'NONE',  ( -0.000000000000000000, -1.000000000000000000, -0.000000000000000000 ) ) ;
#61296=ORIENTED_EDGE ( 'NONE', *, *, #59439, .F. ) ;
#61297=ORIENTED_EDGE ( 'NONE', *, *, #14014, .T. ) ;
#61308=CARTESIAN_POINT ( 'NONE',  ( -6.778443870680312067, -26.22850392868687663, 14.88193859458597856 ) ) ;
#61319=CARTESIAN_POINT ( 'NONE',  ( 11.58535936493820273, -28.03978107659456498, 13.63905399333220281 ) ) ;
#61358=CARTESIAN_POINT ( 'NONE',  ( 16.10228578084485562, -34.99999999976227372, -4.568518662555822729 ) ) ;
#61403=DIRECTION ( 'NONE',  ( 0.000000000000000000, -1.000000000000000000, 0.000000000000000000 ) ) ;
#61413=CARTESIAN_POINT ( 'NONE',  ( -25.00000000000000355, -9.999999999999998224, 5.000000000000002665 ) ) ;
#61424=DIRECTION ( 'NONE',  ( -1.000000000000000000, -0.000000000000000000, -0.000000000000000000 ) ) ;
#61474=CARTESIAN_POINT ( 'NONE',  ( -48.84424248505261090, -0.2332870993691606720, 3.158587530951954658 ) ) ;
#61488=CARTESIAN_POINT ( 'NONE',  ( 18.79103332550323913, -28.91360719445345140, 6.866334764117086209 ) ) ;
#61510=CARTESIAN_POINT ( 'NONE',  ( 19.42209513767211249, -29.99999999999998934, 5.494601501491730211 ) ) ;
#61532=CARTESIAN_POINT ( 'NONE',  ( 48.84659035979348829, -0.2326159177123071076, 2.738175293146158928 ) ) ;
#61538=ORIENTED_EDGE ( 'NONE', *, *, #65363, .F. ) ;
#61549=CARTESIAN_POINT ( 'NONE',  ( 12.39041149895467875, -29.91764912108168417, -8.475516454291387447 ) ) ;
#61578=AXIS2_PLACEMENT_3D ( 'NONE', #13247, #22906, #43159 ) ;
#61584=ORIENTED_EDGE ( 'NONE', *, *, #29951, .T. ) ;
#61598=CARTESIAN_POINT ( 'NONE',  ( 4.308196110052892319E-12, -30.53649492335491189, 15.30974548841782656 ) ) ;
#61603=DIRECTION ( 'NONE',  ( 0.000000000000000000, 1.000000000000000000, 0.000000000000000000 ) ) ;
#61621=VERTEX_POINT ( 'NONE', #28252 ) ;
#61622=DIRECTION ( 'NONE',  ( 0.000000000000000000, 1.000000000000000000, 0.000000000000000000 ) ) ;
#61629=CARTESIAN_POINT ( 'NONE',  ( 4.699914177767785084, -28.11199977926868598, 11.88398404624164506 ) ) ;
#61639=DIRECTION ( 'NONE',  ( 0.000000000000000000, 1.000000000000000000, 0.000000000000000000 ) ) ;
#61768=VECTOR ( 'NONE', #44725, 1000.000000000000000 ) ;
#61782=B_SPLINE_CURVE_WITH_KNOTS ( 'NONE', 3,
 ( #7938, #28207, #6495, #22781, #52388, #31739, #11787, #32068 ),
 .UNSPECIFIED., .F., .F.,
 ( 4, 2, 2, 4 ),
 ( 0.01146705142166408453, 0.01597709677061665001, 0.01823211944509292928, 0.02048714211956921202 ),
 .UNSPECIFIED. ) ;
#61810=CARTESIAN_POINT ( 'NONE',  ( -12.82483530079958989, -29.99871789793482435, -7.856364084349718446 ) ) ;
#61824=CARTESIAN_POINT ( 'NONE',  ( -16.73721172569806015, -28.43318523521388741, 9.619723400408263458 ) ) ;
#61830=CARTESIAN_POINT ( 'NONE',  ( 25.00000000000000355, -9.999999999999998224, 25.00000000000000000 ) ) ;
#61835=CYLINDRICAL_SURFACE ( 'NONE', #40604, 19.00000000000000000 ) ;
#61847=PRESENTATION_STYLE_ASSIGNMENT (( #40243 ) ) ;
#61852=ORIENTED_EDGE ( 'NONE', *, *, #17758, .T. ) ;
#61874=CARTESIAN_POINT ( 'NONE',  ( 26.58564210842044773, -3.638521970294203101, -24.00000000000000711 ) ) ;
#61878=ORIENTED_EDGE ( 'NONE', *, *, #59595, .F. ) ;
#61888=CARTESIAN_POINT ( 'NONE',  ( 37.25000000000000711, -27.56175630915211627, -1.528111002209141978 ) ) ;
#61892=CARTESIAN_POINT ( 'NONE',  ( 8.372133460183917464, -31.76502814486181592, -13.66429824708577812 ) ) ;
#61900=CARTESIAN_POINT ( 'NONE',  ( -10.63305928497607411, -33.14245637257592847, 11.52579945308272968 ) ) ;
#61912=CARTESIAN_POINT ( 'NONE',  ( 41.00000000000000711, 5.493969937218003549E-16, -4.500000000000000888 ) ) ;
#61929=DIRECTION ( 'NONE',  ( 0.000000000000000000, 0.000000000000000000, -1.000000000000000000 ) ) ;
#61955=ORIENTED_EDGE ( 'NONE', *, *, #63965, .T. ) ;
#61976=CARTESIAN_POINT ( 'NONE',  ( 2.990024434114437302, -31.21813892570122206, 14.24440799104838717 ) ) ;
#62098=AXIS2_PLACEMENT_3D ( 'NONE', #57070, #26801, #17808 ) ;
#62119=DIRECTION ( 'NONE',  ( 0.000000000000000000, 1.000000000000000000, 0.000000000000000000 ) ) ;
#62169=CARTESIAN_POINT ( 'NONE',  ( -25.00000000000000355, -9.999999999999998224, -5.000000000000000888 ) ) ;
#62180=CARTESIAN_POINT ( 'NONE',  ( 12.41715713833625401, -27.32744910944862937, -12.80873342738428988 ) ) ;
#62181=CARTESIAN_POINT ( 'NONE',  ( 19.56743653832047514, -30.00000000000000000, 5.000000000000000888 ) ) ;
#62188=CARTESIAN_POINT ( 'NONE',  ( 8.434373009623573836, -31.78234095107705670, -13.63772037845195939 ) ) ;
#62198=CARTESIAN_POINT ( 'NONE',  ( 48.84424248505259669, -0.2332870993691684991, -3.158587530951941780 ) ) ;
#62215=CARTESIAN_POINT ( 'NONE',  ( 17.05023968204111284, -34.49999999999999289, -4.356789313881303194 ) ) ;
#62225=CARTESIAN_POINT ( 'NONE',  ( -16.21117406328131949, -35.00000000000000000, 4.142385751841757724 ) ) ;
#62249=DIRECTION ( 'NONE',  ( 0.000000000000000000, 0.000000000000000000, 1.000000000000000000 ) ) ;
#62271=ORIENTED_EDGE ( 'NONE', *, *, #33875, .F. ) ;
#62284=LINE ( 'NONE', #22056, #1234 ) ;
#62285=CARTESIAN_POINT ( 'NONE',  ( -2.647174210752905488, -25.80125502049867947, 15.55106108913133767 ) ) ;
#62330=EDGE_LOOP ( 'NONE', ( #6224, #55335, #42870, #40804 ) ) ;
#62366=DIRECTION ( 'NONE',  ( -1.000000000000000000, 0.000000000000000000, 0.000000000000000000 ) ) ;
#62383=DIRECTION ( 'NONE',  ( 1.000000000000000000, -0.000000000000000000, 0.000000000000000000 ) ) ;
#62428=DIRECTION ( 'NONE',  ( 1.000000000000000000, -0.000000000000000000, 0.000000000000000000 ) ) ;
#62452=CARTESIAN_POINT ( 'NONE',  ( -17.05023968204110574, -34.50000000000000000, -4.356789313881320957 ) ) ;
#62477=CARTESIAN_POINT ( 'NONE',  ( -19.56743653832046803, -30.00000000000000000, -5.000000000000000888 ) ) ;
#62512=DIRECTION ( 'NONE',  ( -1.000000000000000000, 0.000000000000000000, -0.000000000000000000 ) ) ;
#62528=CARTESIAN_POINT ( 'NONE',  ( 18.18435566811113446, -29.77699652454512957, -8.006764386360391228 ) ) ;
#62538=DIRECTION ( 'NONE',  ( -0.9688695217174484453, 0.000000000000000000, 0.2475719085175105139 ) ) ;
#62545=CONICAL_SURFACE ( 'NONE', #33886, 14.13397459621556251, 0.5235987755983000369 ) ;
#62603=CARTESIAN_POINT ( 'NONE',  ( 10.20102756488484275, -26.83656875578374112, 13.80782716569073010 ) ) ;
#62652=CARTESIAN_POINT ( 'NONE',  ( 4.037157412408303976E-12, -31.03649492335491544, 14.44372008463339085 ) ) ;
#62695=CARTESIAN_POINT ( 'NONE',  ( -47.45484198363494954, -0.5059748548177152028, 8.508429091481763962 ) ) ;
#62726=EDGE_LOOP ( 'NONE', ( #29995, #31557, #43000, #32861 ) ) ;
#62786=CARTESIAN_POINT ( 'NONE',  ( -15.07969093506323865, -34.00054679314069972, -8.511206496388529885 ) ) ;
#62842=AXIS2_PLACEMENT_3D ( 'NONE', #13605, #55492, #65449 ) ;
#62876=CARTESIAN_POINT ( 'NONE',  ( 13.23110845409921055, -34.10188054478342679, -9.409930202775637298 ) ) ;
#62917=CARTESIAN_POINT ( 'NONE',  ( 0.000000000000000000, -34.50000000000000000, 0.000000000000000000 ) ) ;
#62932=CARTESIAN_POINT ( 'NONE',  ( -22.00000000000000711, -20.00000000000000000, 1.500000000000002887 ) ) ;
#62941=ORIENTED_EDGE ( 'NONE', *, *, #45484, .F. ) ;
#62946=ORIENTED_EDGE ( 'NONE', *, *, #35252, .F. ) ;
#62949=CARTESIAN_POINT ( 'NONE',  ( 4.286683309450310730, -28.06227586351137759, 12.00609810331033067 ) ) ;
#62986=CIRCLE ( 'NONE', #9922, 250.0000000000000000 ) ;
#62989=LINE ( 'NONE', #27738, #38631 ) ;
#62996=VERTEX_POINT ( 'NONE', #39118 ) ;
#63021=FACE_OUTER_BOUND ( 'NONE', #7205, .T. ) ;
#63036=CARTESIAN_POINT ( 'NONE',  ( -13.57005631242150834, -30.10739101144227803, 6.607437777793664146 ) ) ;
#63039=CARTESIAN_POINT ( 'NONE',  ( -25.00000000000000355, -3.797884998337192286, 23.99999999999999289 ) ) ;
#63055=LINE ( 'NONE', #36802, #58189 ) ;
#63068=AXIS2_PLACEMENT_3D ( 'NONE', #19214, #14213, #38851 ) ;
#63092=CARTESIAN_POINT ( 'NONE',  ( -12.26308380404417164, -33.73908083898199806, -10.29207979367737380 ) ) ;
#63125=CARTESIAN_POINT ( 'NONE',  ( -16.02805653289969356, -29.20913999211483514, -10.57890313540256777 ) ) ;
#63144=DIRECTION ( 'NONE',  ( -0.9688695217174487784, 0.000000000000000000, -0.2475719085175095702 ) ) ;
#63160=CARTESIAN_POINT ( 'NONE',  ( -17.07517663476617287, -28.52001404462332346, -9.261390606240931689 ) ) ;
#63190=CYLINDRICAL_SURFACE ( 'NONE', #63846, 1.500000000000000444 ) ;
#63196=ORIENTED_EDGE ( 'NONE', *, *, #38142, .F. ) ;
#63201=ORIENTED_EDGE ( 'NONE', *, *, #7030, .T. ) ;
#63209=CARTESIAN_POINT ( 'NONE',  ( 8.006888830052231398, -32.29065697289608750, -12.88904745434341947 ) ) ;
#63212=CARTESIAN_POINT ( 'NONE',  ( 37.25000000000000711, -1.694065894508600678E-18, 0.000000000000000000 ) ) ;
#63215=ORIENTED_EDGE ( 'NONE', *, *, #19492, .T. ) ;
#63228=DIRECTION ( 'NONE',  ( -1.000000000000000000, 0.000000000000000000, 0.000000000000000000 ) ) ;
#63265=CARTESIAN_POINT ( 'NONE',  ( -19.56743653832047514, -33.00000000000000000, -5.000000000000001776 ) ) ;
#63281=ADVANCED_FACE ( 'NONE', ( #47409 ), #36430, .F. ) ;
#63300=AXIS2_PLACEMENT_3D ( 'NONE', #47970, #47324, #17713 ) ;
#63338=DIRECTION ( 'NONE',  ( -0.000000000000000000, 0.000000000000000000, -1.000000000000000000 ) ) ;
#63355=CARTESIAN_POINT ( 'NONE',  ( -48.06591103469482817, -0.3868811097602570803, 6.642178517338849453 ) ) ;
#63369=CARTESIAN_POINT ( 'NONE',  ( -37.25000000000000711, -27.56270118634207833, 0.7455576661145032480 ) ) ;
#63403=CARTESIAN_POINT ( 'NONE',  ( -14.91771861688918399, -27.95837112815216230, -11.21176701200369763 ) ) ;
#63468=CARTESIAN_POINT ( 'NONE',  ( 25.00000000000000355, -9.999999999999998224, 5.000000000000002665 ) ) ;
#63487=CARTESIAN_POINT ( 'NONE',  ( -3.683412895334400528, -30.77133338175680777, 15.02788192793085109 ) ) ;
#63493=LINE ( 'NONE', #22965, #22639 ) ;
#63540=ORIENTED_EDGE ( 'NONE', *, *, #57829, .F. ) ;
#63555=CARTESIAN_POINT ( 'NONE',  ( 3.527934398658575610, -26.69696348912971473, -16.00979375678724637 ) ) ;
#63558=VECTOR ( 'NONE', #25352, 1000.000000000000000 ) ;
#63589=CARTESIAN_POINT ( 'NONE',  ( 17.02556425888772296, -28.50707051634331890, 9.313930266526256219 ) ) ;
#63619=CARTESIAN_POINT ( 'NONE',  ( 0.000000000000000000, -30.50000000000000000, 0.000000000000000000 ) ) ;
#63632=EDGE_CURVE ( 'NONE', #37233, #11603, #22713, .T. ) ;
#63672=CARTESIAN_POINT ( 'NONE',  ( -2.112161198359963521, -26.60281475960710296, 16.15113466974340639 ) ) ;
#63703=CIRCLE ( 'NONE', #61578, 3.999999999999999112 ) ;
#63718=CARTESIAN_POINT ( 'NONE',  ( -29.10325845542003975, -3.352553978523134415, -24.67444324980779413 ) ) ;
#63727=CARTESIAN_POINT ( 'NONE',  ( -5.876491384319547429, -28.27454061773107696, -11.46433771796954382 ) ) ;
#63737=CARTESIAN_POINT ( 'NONE',  ( -37.25000000000000711, -1.694065894508600678E-18, 0.000000000000000000 ) ) ;
#63774=CARTESIAN_POINT ( 'NONE',  ( 41.00000000000000711, -45.00200000000000244, -4.500000000000000888 ) ) ;
#63791=ORIENTED_EDGE ( 'NONE', *, *, #49447, .F. ) ;
#63797=CARTESIAN_POINT ( 'NONE',  ( -17.71439793346019798, -28.67846309484135858, -8.502197385450024569 ) ) ;
#63806=CIRCLE ( 'NONE', #21330, 20.00000000000000000 ) ;
#63808=CARTESIAN_POINT ( 'NONE',  ( 9.648902782401016509, -32.13880772995998569, -13.06387094876276223 ) ) ;
#63827=CARTESIAN_POINT ( 'NONE',  ( 26.58307969160927087, -3.634951060761374197, 23.96081192854775210 ) ) ;
#63846=AXIS2_PLACEMENT_3D ( 'NONE', #64488, #38231, #59516 ) ;
#63855=CARTESIAN_POINT ( 'NONE',  ( -18.01523681890432371, -28.74990419755712878, 8.100995087731217126 ) ) ;
#63861=CARTESIAN_POINT ( 'NONE',  ( 37.25000000000000711, -27.21021009056489603, 4.499999999999997335 ) ) ;
#63865=ADVANCED_FACE ( 'NONE', ( #57225 ), #26960, .T. ) ;
#63883=EDGE_CURVE ( 'NONE', #33520, #17827, #55766, .T. ) ;
#63897=CARTESIAN_POINT ( 'NONE',  ( 10.75388052849567799, -27.84561629232752011, -14.03224735226135245 ) ) ;
#63933=CARTESIAN_POINT ( 'NONE',  ( 17.33919137821584044, -28.58640580301184286, 8.960163943132222641 ) ) ;
#63940=EDGE_CURVE ( 'NONE', #4569, #2269, #63493, .T. ) ;
#63954=AXIS2_PLACEMENT_3D ( 'NONE', #65551, #54939, #25332 ) ;
#63965=EDGE_CURVE ( 'NONE', #11657, #41367, #43544, .T. ) ;
#64018=CARTESIAN_POINT ( 'NONE',  ( -3.650755842799271012, -28.29207189712390402, 13.56609188631020935 ) ) ;
#64032=ORIENTED_EDGE ( 'NONE', *, *, #57736, .F. ) ;
#64064=CARTESIAN_POINT ( 'NONE',  ( -35.31912638668785576, -2.544741887441773986, -22.78557353984778544 ) ) ;
#64075=CARTESIAN_POINT ( 'NONE',  ( -6.714735010819111949, -31.93429545817926751, -13.37736225704815141 ) ) ;
#64109=EDGE_LOOP ( 'NONE', ( #53794, #65646, #10285, #9562 ) ) ;
#64196=UNCERTAINTY_MEASURE_WITH_UNIT (LENGTH_MEASURE( 1.000000000000000082E-05 ), #50125, 'distance_accuracy_value', 'NONE');
#64219=VERTEX_POINT ( 'NONE', #56486 ) ;
#64230=CARTESIAN_POINT ( 'NONE',  ( 15.74859868605383717, -29.13321728093753649, -10.87107032828078701 ) ) ;
#64248=AXIS2_PLACEMENT_3D ( 'NONE', #37680, #47654, #2100 ) ;
#64281=ORIENTED_EDGE ( 'NONE', *, *, #44360, .F. ) ;
#64327=CARTESIAN_POINT ( 'NONE',  ( -38.57634030218385846, -26.62784119520750892, 4.499999999999997335 ) ) ;
#64334=EDGE_CURVE ( 'NONE', #7333, #52741, #49782, .T. ) ;
#64341=CARTESIAN_POINT ( 'NONE',  ( -16.37486794060187734, -29.30468282063785779, 10.24044889374758149 ) ) ;
#64387=CARTESIAN_POINT ( 'NONE',  ( 4.682340427901537261, -31.48164499408211014, -13.94155213824621953 ) ) ;
#64440=CARTESIAN_POINT ( 'NONE',  ( 0.000000000000000000, -30.50000000000000000, 0.000000000000000000 ) ) ;
#64449=EDGE_CURVE ( 'NONE', #29328, #23145, #62989, .T. ) ;
#64488=CARTESIAN_POINT ( 'NONE',  ( -22.00000000000000711, -20.00000000000000000, 2.449293598294706907E-15 ) ) ;
#64508=CARTESIAN_POINT ( 'NONE',  ( -15.09490394635370336, -34.00569493827350698, -8.490101771330714087 ) ) ;
#64514=CARTESIAN_POINT ( 'NONE',  ( 38.57634030218385846, -26.62784119520750892, 4.499999999999997335 ) ) ;
#64539=CARTESIAN_POINT ( 'NONE',  ( -14.99915657824959325, -28.92607294587373090, -11.47448459775364604 ) ) ;
#64590=ORIENTED_EDGE ( 'NONE', *, *, #24570, .T. ) ;
#64609=ORIENTED_EDGE ( 'NONE', *, *, #5223, .T. ) ;
#64635=EDGE_LOOP ( 'NONE', ( #49672, #32281, #12567, #58453 ) ) ;
#64649=DIRECTION ( 'NONE',  ( -1.000000000000000000, -0.000000000000000000, -0.000000000000000000 ) ) ;
#64654=CARTESIAN_POINT ( 'NONE',  ( 3.702144525957873356, -26.71142515285348651, 15.98786919972943288 ) ) ;
#64704=CARTESIAN_POINT ( 'NONE',  ( -5.261125060311115931, -26.02247534669140094, -15.21511059005040423 ) ) ;
#64724=ORIENTED_EDGE ( 'NONE', *, *, #3123, .F. ) ;
#64738=ORIENTED_EDGE ( 'NONE', *, *, #1799, .F. ) ;
#64767=VERTEX_POINT ( 'NONE', #1357 ) ;
#64774=DIRECTION ( 'NONE',  ( 0.000000000000000000, 1.000000000000000000, 0.000000000000000000 ) ) ;
#64803=AXIS2_PLACEMENT_3D ( 'NONE', #28759, #49073, #43061 ) ;
#64807=DIRECTION ( 'NONE',  ( 0.000000000000000000, -0.000000000000000000, 1.000000000000000000 ) ) ;
#64810=AXIS2_PLACEMENT_3D ( 'NONE', #12454, #32726, #48400 ) ;
#64854=CARTESIAN_POINT ( 'NONE',  ( -16.12286248669609634, -29.23548504417003713, 10.48934106169928704 ) ) ;
#64874=EDGE_CURVE ( 'NONE', #15355, #18319, #16374, .T. ) ;
#64900=CARTESIAN_POINT ( 'NONE',  ( -7.049735699849408732, -28.78059498260830651, -12.46475915493682152 ) ) ;
#64931=ADVANCED_FACE ( 'NONE', ( #54457 ), #3606, .T. ) ;
#64945=CARTESIAN_POINT ( 'NONE',  ( 40.19089168456218175, -1.800105668799817593, -19.87241647152735169 ) ) ;
#64993=CARTESIAN_POINT ( 'NONE',  ( -6.778443870680312067, -27.08263571440717854, 15.40204062588007616 ) ) ;
#65020=FACE_OUTER_BOUND ( 'NONE', #49948, .T. ) ;
#65035=CARTESIAN_POINT ( 'NONE',  ( -6.008663266769909583, -31.76136623419866822, -13.60005156547899041 ) ) ;
#65041=CARTESIAN_POINT ( 'NONE',  ( -6.641947195041168150, -28.39580239767160919, -11.12859478088952336 ) ) ;
#65065=ORIENTED_EDGE ( 'NONE', *, *, #5727, .T. ) ;
#65103=VECTOR ( 'NONE', #50127, 1000.000000000000000 ) ;
#65117=VECTOR ( 'NONE', #20224, 1000.000000000000000 ) ;
#65148=EDGE_CURVE ( 'NONE', #38736, #37992, #1551, .T. ) ;
#65149=VECTOR ( 'NONE', #24175, 1000.000000000000000 ) ;
#65150=VERTEX_POINT ( 'NONE', #7836 ) ;
#65161=FACE_OUTER_BOUND ( 'NONE', #33561, .T. ) ;
#65164=EDGE_LOOP ( 'NONE', ( #7601, #45851, #30890, #54353 ) ) ;
#65178=CARTESIAN_POINT ( 'NONE',  ( -1.318817192132426526E-11, -30.53649492335491544, -15.30974548841782834 ) ) ;
#65180=FACE_OUTER_BOUND ( 'NONE', #33178, .T. ) ;
#65211=CARTESIAN_POINT ( 'NONE',  ( -5.041025311761536898, -26.84022127302798921, -15.79220748139830910 ) ) ;
#65235=CARTESIAN_POINT ( 'NONE',  ( 25.00000000000000355, -9.999999999999998224, 1.530808498934191521E-15 ) ) ;
#65244=CARTESIAN_POINT ( 'NONE',  ( -7.278994278378523752, -27.16225867570108932, -15.27062364585639287 ) ) ;
#65286=CARTESIAN_POINT ( 'NONE',  ( 48.66712064925836501, -0.2684213679329396918, -8.095633725969733518 ) ) ;
#65292=CARTESIAN_POINT ( 'NONE',  ( 0.9207726606957047366, -30.53649492335506466, 15.30974548841765426 ) ) ;
#65296=FACE_OUTER_BOUND ( 'NONE', #51027, .T. ) ;
#65316=CARTESIAN_POINT ( 'NONE',  ( -11.13200843151504849, -27.03228069553586010, 13.43438493493725616 ) ) ;
#65326=CARTESIAN_POINT ( 'NONE',  ( 13.98043512791166698, -30.12632228061958273, 5.689268883804715848 ) ) ;
#65346=ORIENTED_EDGE ( 'NONE', *, *, #14014, .F. ) ;
#65363=EDGE_CURVE ( 'NONE', #53403, #22226, #12125, .T. ) ;
#65364=CARTESIAN_POINT ( 'NONE',  ( -3.498383876438375228, -31.27426290440411094, -14.18200193795731145 ) ) ;
#65369=CARTESIAN_POINT ( 'NONE',  ( 12.91449914267798960, -27.44768092100439461, -12.53791341943762916 ) ) ;
#65376=AXIS2_PLACEMENT_3D ( 'NONE', #42577, #41940, #62538 ) ;
#65391=CARTESIAN_POINT ( 'NONE',  ( 25.00000000000000355, -30.00000000000000000, 24.00000000000000000 ) ) ;
#65408=DIRECTION ( 'NONE',  ( 0.000000000000000000, 1.000000000000000000, 0.000000000000000000 ) ) ;
#65419=CARTESIAN_POINT ( 'NONE',  ( 19.56743653832046803, -33.00000000000000000, -5.000000000000012434 ) ) ;
#65449=DIRECTION ( 'NONE',  ( 0.000000000000000000, 0.000000000000000000, 1.000000000000000000 ) ) ;
#65506=SURFACE_STYLE_FILL_AREA ( #45250 ) ;
#65535=EDGE_LOOP ( 'NONE', ( #23612, #63791 ) ) ;
#65539=CIRCLE ( 'NONE', #53904, 17.19615242270663558 ) ;
#65547=CARTESIAN_POINT ( 'NONE',  ( -2.647174210752900603, -26.63290002157760128, -16.10638009382239488 ) ) ;
#65551=CARTESIAN_POINT ( 'NONE',  ( 0.000000000000000000, -30.00000000000000000, 0.000000000000000000 ) ) ;
#65588=EDGE_CURVE ( 'NONE', #60939, #33165, #41898, .T. ) ;
#65591=CARTESIAN_POINT ( 'NONE',  ( 43.82484328533828233, -1.182663722159852604, 16.53294353590085208 ) ) ;
#65593=CARTESIAN_POINT ( 'NONE',  ( -41.49302228377220558, -1.586477970524134085, -18.85982933713411214 ) ) ;
#65603=CARTESIAN_POINT ( 'NONE',  ( 25.00000000000000355, -9.999999999999998224, 1.530808498934191521E-15 ) ) ;
#65631=CARTESIAN_POINT ( 'NONE',  ( 8.617947477504868559, -29.08580380500490747, 11.66524603227121659 ) ) ;
#65640=CIRCLE ( 'NONE', #29526, 1.500000000000000444 ) ;
#65646=ORIENTED_EDGE ( 'NONE', *, *, #9872, .F. ) ;
#65661=CARTESIAN_POINT ( 'NONE',  ( 37.25000000000000711, -45.00200000000000244, -4.500000000000000888 ) ) ;
#65682=CARTESIAN_POINT ( 'NONE',  ( 15.64085769076060295, -34.91570230176446898, -5.822163132929507157 ) ) ;
#65701=CARTESIAN_POINT ( 'NONE',  ( -25.00000000000000355, -30.00000000000000000, 25.00000000000000000 ) ) ;
#65704=VERTEX_POINT ( 'NONE', #35623 ) ;
#65805=CARTESIAN_POINT ( 'NONE',  ( 17.05919086487388370, -28.51594916623512432, 9.278936603800783445 ) ) ;
ENDSEC;
END-ISO-10303-21;
